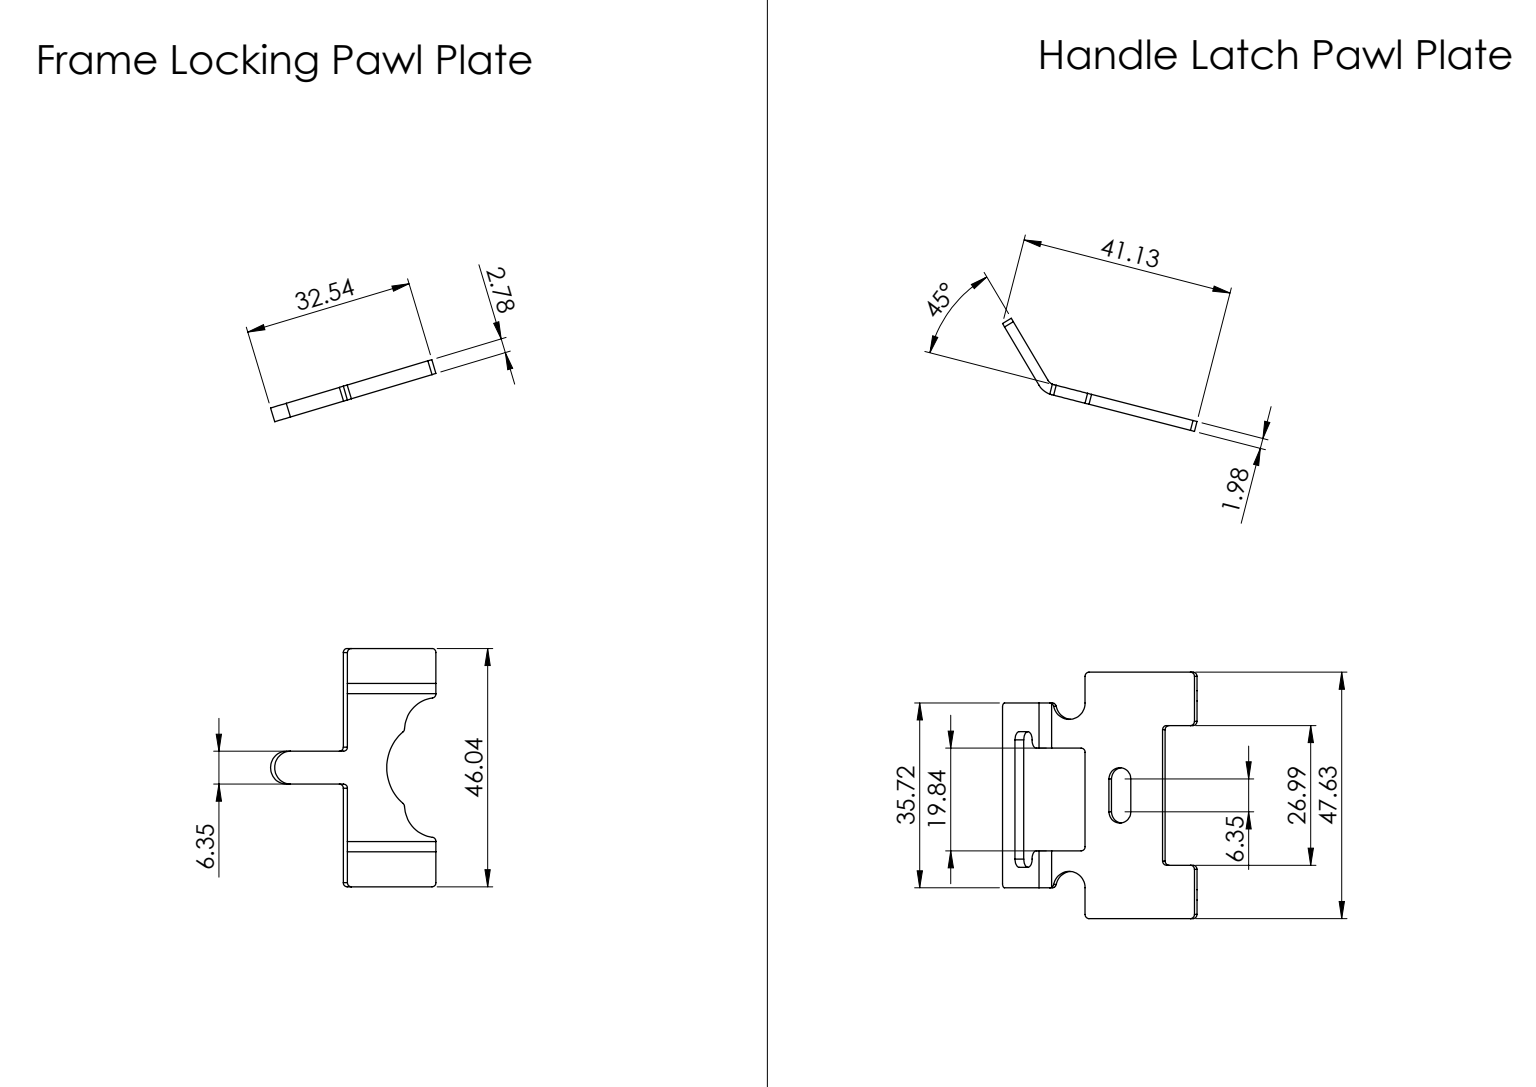
ISO-10303-21;
HEADER;
FILE_DESCRIPTION (('STEP AP214'),
    '1' );
FILE_NAME ('Handle Latch Pawl Plate.step',
    '2026-10-09T14:10:49',
    ( '' ),
    ( '' ),
    'SwSTEP 2.0',
    'SolidWorks 2026',
    '' );
FILE_SCHEMA (( 'AUTOMOTIVE_DESIGN' ));
ENDSEC;

DATA;
#10=CARTESIAN_POINT ( 'NONE',  ( 24.26606285357373594, 2.770822500000000854, -16.92219937337620195 ) ) ;
#13=VECTOR ( 'NONE', #12201, 1000.000000000000000 ) ;
#33=SHAPE_REPRESENTATION_RELATIONSHIP ( 'NONE' , 'NONE' ,  #560, #17207 ) ;
#39=CARTESIAN_POINT ( 'NONE',  ( -0.5435003404963313356, 2.373947500000000765, -25.80650133522849998 ) ) ;
#48=DIRECTION ( 'NONE',  ( 0.000000000000000000, -1.000000000000000000, 0.000000000000000000 ) ) ;
#49=ORIENTED_EDGE ( 'NONE', *, *, #10493, .T. ) ;
#66=ORIENTED_EDGE ( 'NONE', *, *, #20020, .T. ) ;
#83=EDGE_CURVE ( 'NONE', #6123, #21755, #12204, .T. ) ;
#96=DIRECTION ( 'NONE',  ( 0.000000000000000000, 1.000000000000000000, 0.000000000000000000 ) ) ;
#99=VECTOR ( 'NONE', #5317, 1000.000000000000114 ) ;
#111=DIRECTION ( 'NONE',  ( 0.2490110332224850509, 0.000000000000000000, -0.9685006480810792739 ) ) ;
#157=EDGE_CURVE ( 'NONE', #13662, #8452, #17280, .T. ) ;
#167=ADVANCED_FACE ( 'NONE', ( #2245 ), #15977, .T. ) ;
#183=AXIS2_PLACEMENT_3D ( 'NONE', #21265, #19500, #6119 ) ;
#192=CARTESIAN_POINT ( 'NONE',  ( 1.416441012474747074, 34.09397655050049991, -20.74814719358345627 ) ) ;
#195=DIRECTION ( 'NONE',  ( 0.000000000000000000, 1.000000000000000000, 0.000000000000000000 ) ) ;
#203=EDGE_CURVE ( 'NONE', #6199, #19184, #15619, .T. ) ;
#215=CARTESIAN_POINT ( 'NONE',  ( 4.520836821130160388, 5.548947500000001476, -5.476444653012091379 ) ) ;
#222=PLANE ( 'NONE',  #19482 ) ;
#237=EDGE_CURVE ( 'NONE', #10280, #1619, #6209, .T. ) ;
#244=DIRECTION ( 'NONE',  ( 0.8609107660235850723, 0.000000000000000000, -0.5087559856598092844 ) ) ;
#263=ORIENTED_EDGE ( 'NONE', *, *, #13066, .F. ) ;
#272=EDGE_CURVE ( 'NONE', #13945, #11658, #11090, .T. ) ;
#300=DIRECTION ( 'NONE',  ( -0.5087559856598092844, -0.000000000000000000, -0.8609107660235850723 ) ) ;
#308=FACE_OUTER_BOUND ( 'NONE', #12169, .T. ) ;
#318=ORIENTED_EDGE ( 'NONE', *, *, #7660, .F. ) ;
#328=DIRECTION ( 'NONE',  ( -0.2490110332224850509, 0.000000000000000000, 0.9685006480810792739 ) ) ;
#361=CARTESIAN_POINT ( 'NONE',  ( 14.73791976308111451, 13.08957250000000094, -17.32306410839158772 ) ) ;
#372=AXIS2_PLACEMENT_3D ( 'NONE', #2270, #15784, #5467 ) ;
#399=AXIS2_PLACEMENT_3D ( 'NONE', #8708, #17541, #7472 ) ;
#408=CARTESIAN_POINT ( 'NONE',  ( 1.923689137428217455, -0.9589899600121986056, -20.61772871637841220 ) ) ;
#410=VECTOR ( 'NONE', #17472, 1000.000000000000114 ) ;
#415=CARTESIAN_POINT ( 'NONE',  ( -6.268352501591477832, 33.32892749999999893, -35.49402737582407497 ) ) ;
#420=VECTOR ( 'NONE', #6179, 1000.000000000000114 ) ;
#425=EDGE_LOOP ( 'NONE', ( #3626, #10707, #4614, #14152, #12802, #17035 ) ) ;
#431=VECTOR ( 'NONE', #2432, 1000.000000000000114 ) ;
#435=CARTESIAN_POINT ( 'NONE',  ( 28.87608719841374949, 1.975802500000001904, -15.73691681567849976 ) ) ;
#457=ORIENTED_EDGE ( 'NONE', *, *, #18854, .F. ) ;
#462=AXIS2_PLACEMENT_3D ( 'NONE', #21471, #19700, #9852 ) ;
#474=DIRECTION ( 'NONE',  ( 0.2490110332224850231, 0.000000000000000000, -0.9685006480810791629 ) ) ;
#475=CARTESIAN_POINT ( 'NONE',  ( 29.64606458365116737, -7.547927499999999235, -15.53894806404596096 ) ) ;
#478=EDGE_CURVE ( 'NONE', #18112, #12175, #19125, .T. ) ;
#480=ORIENTED_EDGE ( 'NONE', *, *, #17479, .T. ) ;
#490=VERTEX_POINT ( 'NONE', #7825 ) ;
#492=EDGE_CURVE ( 'NONE', #3590, #2498, #6272, .T. ) ;
#508=CARTESIAN_POINT ( 'NONE',  ( 19.07578797920377411, 34.51447250000000366, -18.25667004382573566 ) ) ;
#510=FACE_OUTER_BOUND ( 'NONE', #6893, .T. ) ;
#513=VERTEX_POINT ( 'NONE', #11150 ) ;
#514=DIRECTION ( 'NONE',  ( -0.9685006480810792739, 0.000000000000000000, -0.2490110332224850509 ) ) ;
#517=CARTESIAN_POINT ( 'NONE',  ( 1.670997140563193373, 34.12394749999999988, -22.76294857149378714 ) ) ;
#526=CARTESIAN_POINT ( 'NONE',  ( 1.998220421679061776, 25.39269750000000059, -22.64748046904500356 ) ) ;
#547=DIRECTION ( 'NONE',  ( 0.000000000000000000, 1.000000000000000000, 0.000000000000000000 ) ) ;
#560=SHAPE_REPRESENTATION ( 'Handle Latch Pawl Plate', ( #2234 ), #14439 ) ;
#565=PLANE ( 'NONE',  #6360 ) ;
#578=CARTESIAN_POINT ( 'NONE',  ( -5.536601939709260733, 3.961447500000001565, -30.39452380949970944 ) ) ;
#593=AXIS2_PLACEMENT_3D ( 'NONE', #12095, #15316, #1903 ) ;
#594=CARTESIAN_POINT ( 'NONE',  ( -6.268352501600194415, -1.265494433635971250, -35.49402737582123990 ) ) ;
#631=ORIENTED_EDGE ( 'NONE', *, *, #14864, .T. ) ;
#635=CARTESIAN_POINT ( 'NONE',  ( 7.735533989518945219, 5.548947500000001476, -21.17236077523805449 ) ) ;
#645=VECTOR ( 'NONE', #6896, 1000.000000000000114 ) ;
#647=CARTESIAN_POINT ( 'NONE',  ( 19.07578797920376701, -3.966527499999997097, -18.25667004382573921 ) ) ;
#663=ORIENTED_EDGE ( 'NONE', *, *, #15860, .F. ) ;
#670=CARTESIAN_POINT ( 'NONE',  ( 1.776692311944953584, 34.12394749999999988, -22.71488278333200839 ) ) ;
#720=CIRCLE ( 'NONE', #9536, 0.7950200000000005041 ) ;
#727=ORIENTED_EDGE ( 'NONE', *, *, #2466, .F. ) ;
#732=LINE ( 'NONE', #7593, #11396 ) ;
#750=EDGE_LOOP ( 'NONE', ( #6315, #10700, #9277, #2077, #19066, #6524 ) ) ;
#754=AXIS2_PLACEMENT_3D ( 'NONE', #7235, #13993, #4124 ) ;
#762=ADVANCED_FACE ( 'NONE', ( #16785 ), #13268, .T. ) ;
#788=AXIS2_PLACEMENT_3D ( 'NONE', #5490, #4369, #1956 ) ;
#794=DIRECTION ( 'NONE',  ( -0.000000000000000000, 1.000000000000000000, 0.000000000000000000 ) ) ;
#805=VECTOR ( 'NONE', #14773, 1000.000000000000114 ) ;
#808=EDGE_LOOP ( 'NONE', ( #8099, #12394, #12847, #19398, #3996, #13078 ) ) ;
#839=DIRECTION ( 'NONE',  ( 0.8558687090795832342, 0.000000000000000000, -0.5171931484643309540 ) ) ;
#871=CIRCLE ( 'NONE', #6171, 3.174999999999998490 ) ;
#875=CARTESIAN_POINT ( 'NONE',  ( 2.492193568723835462, -69.63187750000000165, -24.56873394466936134 ) ) ;
#879=CARTESIAN_POINT ( 'NONE',  ( -1.427050033073577806, 5.548947500000001476, -23.44038945102687066 ) ) ;
#884=ORIENTED_EDGE ( 'NONE', *, *, #3946, .T. ) ;
#892=FACE_OUTER_BOUND ( 'NONE', #17084, .T. ) ;
#903=CARTESIAN_POINT ( 'NONE',  ( -23.36909032872569014, 3.961447500000001565, -10.47372115209112842 ) ) ;
#911=EDGE_LOOP ( 'NONE', ( #2038, #5013, #2441, #3955 ) ) ;
#942=DIRECTION ( 'NONE',  ( 0.000000000000000000, -1.000000000000000000, 0.000000000000000000 ) ) ;
#946=PLANE ( 'NONE',  #19198 ) ;
#992=EDGE_CURVE ( 'NONE', #20634, #7630, #3840, .T. ) ;
#999=CARTESIAN_POINT ( 'NONE',  ( 28.38195592936287781, -6.752907499999998286, -13.81504834214261024 ) ) ;
#1000=DIRECTION ( 'NONE',  ( -0.000000000000000000, 1.000000000000000000, 0.000000000000000000 ) ) ;
#1001=DIRECTION ( 'NONE',  ( 0.2490110332224850231, 0.000000000000000000, -0.9685006480810791629 ) ) ;
#1013=VECTOR ( 'NONE', #20361, 1000.000000000000114 ) ;
#1047=ORIENTED_EDGE ( 'NONE', *, *, #11652, .T. ) ;
#1048=LINE ( 'NONE', #21490, #15598 ) ;
#1071=DIRECTION ( 'NONE',  ( 0.9685006480810790519, 0.000000000000000000, 0.2490110332224857170 ) ) ;
#1091=DIRECTION ( 'NONE',  ( 0.000000000000000000, 1.000000000000000000, 0.000000000000000000 ) ) ;
#1093=DIRECTION ( 'NONE',  ( -0.9685006480810791629, 0.000000000000000000, -0.2490110332224850231 ) ) ;
#1096=VERTEX_POINT ( 'NONE', #4892 ) ;
#1134=ORIENTED_EDGE ( 'NONE', *, *, #19533, .F. ) ;
#1150=CARTESIAN_POINT ( 'NONE',  ( 28.38195592936287781, 2.770822500000000854, -13.81504834214261024 ) ) ;
#1154=DIRECTION ( 'NONE',  ( -0.8558687090795832342, 0.000000000000000000, 0.5171931484643309540 ) ) ;
#1180=CARTESIAN_POINT ( 'NONE',  ( 15.23205103213198441, 13.08957250000000094, -19.24493258192747902 ) ) ;
#1194=EDGE_LOOP ( 'NONE', ( #3150, #13135, #19731, #16444 ) ) ;
#1196=DIRECTION ( 'NONE',  ( -0.8609107660235849613, 0.000000000000000000, 0.5087559856598092844 ) ) ;
#1200=DIRECTION ( 'NONE',  ( -0.2490110332224850509, 0.000000000000000000, 0.9685006480810792739 ) ) ;
#1216=VERTEX_POINT ( 'NONE', #20126 ) ;
#1220=EDGE_CURVE ( 'NONE', #9160, #4533, #11757, .T. ) ;
#1267=( NAMED_UNIT ( * ) PLANE_ANGLE_UNIT ( ) SI_UNIT ( $, .RADIAN. ) );
#1281=CARTESIAN_POINT ( 'NONE',  ( -6.268352501604232963, 33.79463943363963807, -35.49402737582801848 ) ) ;
#1282=DIRECTION ( 'NONE',  ( -0.5087559856598092844, 0.000000000000000000, -0.8609107660235849613 ) ) ;
#1290=ADVANCED_FACE ( 'NONE', ( #17049 ), #1896, .T. ) ;
#1295=VERTEX_POINT ( 'NONE', #13752 ) ;
#1336=ADVANCED_FACE ( 'NONE', ( #17716 ), #15964, .T. ) ;
#1355=EDGE_CURVE ( 'NONE', #13546, #14729, #6108, .T. ) ;
#1371=AXIS2_PLACEMENT_3D ( 'NONE', #14359, #9464, #21074 ) ;
#1372=ORIENTED_EDGE ( 'NONE', *, *, #1935, .T. ) ;
#1407=VECTOR ( 'NONE', #1001, 1000.000000000000114 ) ;
#1436=CARTESIAN_POINT ( 'NONE',  ( 9.275488759993784527, 39.28205249999999893, -20.77642327197297689 ) ) ;
#1438=DIRECTION ( 'NONE',  ( -0.3393000355767771259, 0.000000000000000000, 0.9406782052634140578 ) ) ;
#1472=ORIENTED_EDGE ( 'NONE', *, *, #18070, .T. ) ;
#1473=DIRECTION ( 'NONE',  ( 0.000000000000000000, -1.000000000000000000, 0.000000000000000000 ) ) ;
#1480=VERTEX_POINT ( 'NONE', #4310 ) ;
#1484=CIRCLE ( 'NONE', #3603, 1.983740000000000503 ) ;
#1494=CARTESIAN_POINT ( 'NONE',  ( 28.87608719841374949, 29.75832250000000201, -15.73691681567849976 ) ) ;
#1496=VECTOR ( 'NONE', #10087, 1000.000000000000114 ) ;
#1506=DIRECTION ( 'NONE',  ( 0.2490110332224850509, 0.000000000000000000, -0.9685006480810792739 ) ) ;
#1537=ADVANCED_FACE ( 'NONE', ( #4632 ), #2983, .T. ) ;
#1541=ORIENTED_EDGE ( 'NONE', *, *, #4537, .F. ) ;
#1560=EDGE_LOOP ( 'NONE', ( #19520, #15225, #14345, #9159, #6722, #1134 ) ) ;
#1579=LINE ( 'NONE', #11435, #21377 ) ;
#1585=PLANE ( 'NONE',  #593 ) ;
#1601=DIRECTION ( 'NONE',  ( -0.9685006480810791629, 0.000000000000000000, -0.2490110332224850231 ) ) ;
#1612=ORIENTED_EDGE ( 'NONE', *, *, #3894, .T. ) ;
#1619=VERTEX_POINT ( 'NONE', #14609 ) ;
#1632=VERTEX_POINT ( 'NONE', #6178 ) ;
#1645=CARTESIAN_POINT ( 'NONE',  ( -7.949728765564807453, 33.79463943364264367, -34.47798802950575237 ) ) ;
#1646=DIRECTION ( 'NONE',  ( 0.000000000000000000, -1.000000000000000000, 0.000000000000000000 ) ) ;
#1649=CIRCLE ( 'NONE', #18962, 3.970020000000001215 ) ;
#1665=DIRECTION ( 'NONE',  ( -0.5087559856598092844, 0.000000000000000000, -0.8609107660235849613 ) ) ;
#1717=CARTESIAN_POINT ( 'NONE',  ( 11.24737647850577993, 19.43957250000000059, -3.746985211334052046 ) ) ;
#1721=VERTEX_POINT ( 'NONE', #6934 ) ;
#1723=DIRECTION ( 'NONE',  ( 0.000000000000000000, 1.000000000000000000, 0.000000000000000000 ) ) ;
#1740=CARTESIAN_POINT ( 'NONE',  ( 24.26606285357373594, 29.75832250000000201, -16.92219937337620195 ) ) ;
#1757=ORIENTED_EDGE ( 'NONE', *, *, #17479, .F. ) ;
#1762=VERTEX_POINT ( 'NONE', #20081 ) ;
#1766=ORIENTED_EDGE ( 'NONE', *, *, #20682, .F. ) ;
#1782=CARTESIAN_POINT ( 'NONE',  ( 0.2641497867371597752, 26.98019749999999917, -24.43980549416641068 ) ) ;
#1785=B_SPLINE_CURVE_WITH_KNOTS ( 'NONE', 3,
 ( #10743, #10628, #670, #19132 ),
 .UNSPECIFIED., .F., .F.,
 ( 4, 4 ),
 ( 0.000000000000000000, 1.000000000000000000 ),
 .UNSPECIFIED. ) ;
#1804=LINE ( 'NONE', #18606, #19796 ) ;
#1809=ORIENTED_EDGE ( 'NONE', *, *, #492, .F. ) ;
#1840=ORIENTED_EDGE ( 'NONE', *, *, #2050, .F. ) ;
#1864=DIRECTION ( 'NONE',  ( -0.8609107660235848503, 0.000000000000000000, 0.5087559856598096175 ) ) ;
#1865=EDGE_LOOP ( 'NONE', ( #727, #19010, #8001, #1904 ) ) ;
#1869=CARTESIAN_POINT ( 'NONE',  ( 2.520748753591570690, 102.1610225000000014, -24.56335908395234924 ) ) ;
#1874=CARTESIAN_POINT ( 'NONE',  ( -3.042350287543033716, 3.961447500000001565, -26.17378113315171007 ) ) ;
#1875=DIRECTION ( 'NONE',  ( 0.000000000000000000, 1.000000000000000000, 0.000000000000000000 ) ) ;
#1884=CARTESIAN_POINT ( 'NONE',  ( -6.268352501591477832, -7.547927499999999235, -35.49402737582407497 ) ) ;
#1896=PLANE ( 'NONE',  #9972 ) ;
#1903=DIRECTION ( 'NONE',  ( 0.000000000000000000, 1.000000000000000000, 0.000000000000000000 ) ) ;
#1904=ORIENTED_EDGE ( 'NONE', *, *, #10523, .T. ) ;
#1935=EDGE_CURVE ( 'NONE', #19764, #15380, #18870, .T. ) ;
#1938=ORIENTED_EDGE ( 'NONE', *, *, #10853, .F. ) ;
#1952=CARTESIAN_POINT ( 'NONE',  ( 23.77193158452286781, 28.96330250000000461, -15.00033089984030887 ) ) ;
#1956=DIRECTION ( 'NONE',  ( 0.000000000000000000, 1.000000000000000000, 0.000000000000000000 ) ) ;
#1957=DIRECTION ( 'NONE',  ( 0.2490110332224850509, 0.000000000000000000, -0.9685006480810792739 ) ) ;
#1962=ORIENTED_EDGE ( 'NONE', *, *, #7537, .T. ) ;
#1981=VERTEX_POINT ( 'NONE', #15914 ) ;
#2019=DIRECTION ( 'NONE',  ( 0.2490110332224850509, 0.000000000000000000, -0.9685006480810792739 ) ) ;
#2038=ORIENTED_EDGE ( 'NONE', *, *, #2764, .T. ) ;
#2050=EDGE_CURVE ( 'NONE', #21656, #4533, #12134, .T. ) ;
#2061=DIRECTION ( 'NONE',  ( 0.5087559856598092844, 0.000000000000000000, 0.8609107660235849613 ) ) ;
#2077=ORIENTED_EDGE ( 'NONE', *, *, #5527, .F. ) ;
#2078=EDGE_CURVE ( 'NONE', #21155, #5628, #13555, .T. ) ;
#2097=ORIENTED_EDGE ( 'NONE', *, *, #203, .F. ) ;
#2119=CARTESIAN_POINT ( 'NONE',  ( 29.64606458365116737, 34.51447250000000366, -15.53894806404596096 ) ) ;
#2125=CARTESIAN_POINT ( 'NONE',  ( 29.64606458365116737, -6.752907499999998286, -15.53894806404596096 ) ) ;
#2157=ORIENTED_EDGE ( 'NONE', *, *, #21610, .F. ) ;
#2175=CIRCLE ( 'NONE', #10306, 1.983739999999997616 ) ;
#2180=CARTESIAN_POINT ( 'NONE',  ( 29.15193331460030279, 30.55334249999999940, -13.61707959051006966 ) ) ;
#2186=AXIS2_PLACEMENT_3D ( 'NONE', #17579, #18897, #17365 ) ;
#2192=ORIENTED_EDGE ( 'NONE', *, *, #7383, .T. ) ;
#2223=FACE_OUTER_BOUND ( 'NONE', #2461, .T. ) ;
#2234=AXIS2_PLACEMENT_3D ( 'NONE', #14022, #2275, #17644 ) ;
#2239=EDGE_CURVE ( 'NONE', #20753, #11503, #4571, .T. ) ;
#2245=FACE_OUTER_BOUND ( 'NONE', #13627, .T. ) ;
#2250=CARTESIAN_POINT ( 'NONE',  ( 1.291462649553455133, -1.594802499999998124, -20.78637864442906746 ) ) ;
#2263=CARTESIAN_POINT ( 'NONE',  ( 0.7843704457339527591, 25.39269750000000059, -23.55949434567611078 ) ) ;
#2266=AXIS2_PLACEMENT_3D ( 'NONE', #19432, #11373, #9591 ) ;
#2270=CARTESIAN_POINT ( 'NONE',  ( -14.17069798364451927, -1.594802499999999013, -10.28222191653059170 ) ) ;
#2275=DIRECTION ( 'NONE',  ( 0.000000000000000000, 0.000000000000000000, 1.000000000000000000 ) ) ;
#2289=CARTESIAN_POINT ( 'NONE',  ( 2.492193568723835462, -69.63187750000000165, -24.56873394466936134 ) ) ;
#2291=CARTESIAN_POINT ( 'NONE',  ( 1.532169971477637782, 34.03012968715594866, -20.71839214105750315 ) ) ;
#2296=ORIENTED_EDGE ( 'NONE', *, *, #6544, .F. ) ;
#2298=VERTEX_POINT ( 'NONE', #14868 ) ;
#2308=DIRECTION ( 'NONE',  ( -0.9685006480810790519, 0.000000000000000000, -0.2490110332224857170 ) ) ;
#2310=FACE_OUTER_BOUND ( 'NONE', #21323, .T. ) ;
#2318=PLANE ( 'NONE',  #21251 ) ;
#2376=VECTOR ( 'NONE', #10947, 1000.000000000000000 ) ;
#2432=DIRECTION ( 'NONE',  ( -0.5087559856598092844, 0.000000000000000000, -0.8609107660235849613 ) ) ;
#2435=ORIENTED_EDGE ( 'NONE', *, *, #21472, .F. ) ;
#2438=DIRECTION ( 'NONE',  ( 0.5087559856598092844, 0.000000000000000000, 0.8609107660235849613 ) ) ;
#2441=ORIENTED_EDGE ( 'NONE', *, *, #5568, .T. ) ;
#2443=AXIS2_PLACEMENT_3D ( 'NONE', #4092, #7521, #10832 ) ;
#2461=EDGE_LOOP ( 'NONE', ( #884, #4206, #14313, #10118, #4181, #10108, #18999, #16892, #15929, #1766, #8567, #19717, #16820, #19420, #14827, #10153, #7652, #7601, #20757, #17660, #1472, #1047, #8293, #7481, #4823, #18978, #17213, #16162 ) ) ;
#2466=EDGE_CURVE ( 'NONE', #21748, #1981, #7554, .T. ) ;
#2495=VERTEX_POINT ( 'NONE', #9826 ) ;
#2498=VERTEX_POINT ( 'NONE', #19892 ) ;
#2510=DIRECTION ( 'NONE',  ( 0.9685006480810790519, 0.000000000000000000, 0.2490110332224857170 ) ) ;
#2523=AXIS2_PLACEMENT_3D ( 'NONE', #16109, #9012, #7687 ) ;
#2526=ORIENTED_EDGE ( 'NONE', *, *, #18854, .T. ) ;
#2541=CARTESIAN_POINT ( 'NONE',  ( -1.629142294184690698, 34.12394749999999988, -7.057664713974870274 ) ) ;
#2552=DIRECTION ( 'NONE',  ( 0.9685006480810793850, 0.000000000000000000, 0.2490110332224848011 ) ) ;
#2558=VECTOR ( 'NONE', #21534, 1000.000000000000000 ) ;
#2569=DIRECTION ( 'NONE',  ( 0.000000000000000000, 1.000000000000000000, 0.000000000000000000 ) ) ;
#2577=VERTEX_POINT ( 'NONE', #8385 ) ;
#2598=EDGE_CURVE ( 'NONE', #17189, #7442, #7339, .T. ) ;
#2605=VECTOR ( 'NONE', #10573, 1000.000000000000000 ) ;
#2627=DIRECTION ( 'NONE',  ( 0.2490110332224850509, 0.000000000000000000, -0.9685006480810792739 ) ) ;
#2639=EDGE_LOOP ( 'NONE', ( #4484, #9676, #15711, #14242 ) ) ;
#2653=LINE ( 'NONE', #16150, #6790 ) ;
#2663=VECTOR ( 'NONE', #20289, 1000.000000000000000 ) ;
#2685=ORIENTED_EDGE ( 'NONE', *, *, #18562, .F. ) ;
#2718=ORIENTED_EDGE ( 'NONE', *, *, #237, .F. ) ;
#2756=PRESENTATION_STYLE_ASSIGNMENT (( #12949 ) ) ;
#2757=ORIENTED_EDGE ( 'NONE', *, *, #13924, .F. ) ;
#2764=EDGE_CURVE ( 'NONE', #8452, #12517, #10390, .T. ) ;
#2765=ORIENTED_EDGE ( 'NONE', *, *, #19882, .T. ) ;
#2769=AXIS2_PLACEMENT_3D ( 'NONE', #10291, #10413, #18685 ) ;
#2772=DIRECTION ( 'NONE',  ( 0.2490110332224850231, 0.000000000000000000, -0.9685006480810791629 ) ) ;
#2788=EDGE_CURVE ( 'NONE', #1096, #20725, #5083, .T. ) ;
#2791=EDGE_CURVE ( 'NONE', #8452, #7807, #20762, .T. ) ;
#2796=VECTOR ( 'NONE', #4237, 1000.000000000000114 ) ;
#2799=CARTESIAN_POINT ( 'NONE',  ( 24.26606285357373594, 2.770822500000000854, -16.92219937337620195 ) ) ;
#2815=ORIENTED_EDGE ( 'NONE', *, *, #14864, .F. ) ;
#2837=VECTOR ( 'NONE', #474, 1000.000000000000114 ) ;
#2842=ADVANCED_FACE ( 'NONE', ( #12165 ), #5623, .F. ) ;
#2864=AXIS2_PLACEMENT_3D ( 'NONE', #5931, #9034, #1071 ) ;
#2871=ORIENTED_EDGE ( 'NONE', *, *, #992, .F. ) ;
#2883=AXIS2_PLACEMENT_3D ( 'NONE', #361, #12308, #10651 ) ;
#2898=DIRECTION ( 'NONE',  ( 0.000000000000000000, 1.000000000000000000, 0.000000000000000000 ) ) ;
#2903=ORIENTED_EDGE ( 'NONE', *, *, #20412, .T. ) ;
#2933=LINE ( 'NONE', #9660, #12813 ) ;
#2943=VERTEX_POINT ( 'NONE', #13832 ) ;
#2944=AXIS2_PLACEMENT_3D ( 'NONE', #1782, #12081, #20447 ) ;
#2951=AXIS2_PLACEMENT_3D ( 'NONE', #11235, #14800, #2510 ) ;
#2962=ORIENTED_EDGE ( 'NONE', *, *, #11927, .F. ) ;
#2968=AXIS2_PLACEMENT_3D ( 'NONE', #8717, #12385, #2308 ) ;
#2973=AXIS2_PLACEMENT_3D ( 'NONE', #19298, #7264, #12679 ) ;
#2979=DIRECTION ( 'NONE',  ( 0.2490110332224850231, 0.000000000000000000, -0.9685006480810791629 ) ) ;
#2982=ORIENTED_EDGE ( 'NONE', *, *, #5220, .F. ) ;
#2983=CYLINDRICAL_SURFACE ( 'NONE', #7522, 0.7950200000000001710 ) ;
#2994=VERTEX_POINT ( 'NONE', #6273 ) ;
#3000=DIRECTION ( 'NONE',  ( 0.000000000000000000, -1.000000000000000000, 0.000000000000000000 ) ) ;
#3012=ORIENTED_EDGE ( 'NONE', *, *, #478, .T. ) ;
#3039=ORIENTED_EDGE ( 'NONE', *, *, #13022, .F. ) ;
#3058=CARTESIAN_POINT ( 'NONE',  ( -6.268352501591477832, 33.32892749999999893, -35.49402737582407497 ) ) ;
#3075=ORIENTED_EDGE ( 'NONE', *, *, #7315, .F. ) ;
#3088=CARTESIAN_POINT ( 'NONE',  ( 1.998220421679061776, -1.515722362770699494, -22.64748046904500356 ) ) ;
#3111=VERTEX_POINT ( 'NONE', #7826 ) ;
#3119=CARTESIAN_POINT ( 'NONE',  ( 7.735533989518945219, 5.548947500000001476, -21.17236077523805449 ) ) ;
#3122=DIRECTION ( 'NONE',  ( 0.000000000000000000, -1.000000000000000000, 0.000000000000000000 ) ) ;
#3150=ORIENTED_EDGE ( 'NONE', *, *, #11028, .T. ) ;
#3152=ORIENTED_EDGE ( 'NONE', *, *, #21472, .T. ) ;
#3158=LINE ( 'NONE', #15016, #5901 ) ;
#3181=CARTESIAN_POINT ( 'NONE',  ( 24.36723594150488026, 30.55334249999999940, 1.799757394719970982 ) ) ;
#3183=VECTOR ( 'NONE', #48, 1000.000000000000000 ) ;
#3198=DIRECTION ( 'NONE',  ( -0.2490110332224849676, 0.000000000000000000, 0.9685006480810792739 ) ) ;
#3206=DIRECTION ( 'NONE',  ( -0.2490110332224850509, 0.000000000000000000, 0.9685006480810792739 ) ) ;
#3207=AXIS2_PLACEMENT_3D ( 'NONE', #5858, #16163, #5960 ) ;
#3228=CIRCLE ( 'NONE', #20150, 1.983740000000001391 ) ;
#3230=LINE ( 'NONE', #3119, #15881 ) ;
#3231=CARTESIAN_POINT ( 'NONE',  ( 1.169308704210513694, 33.32892749999999893, -20.81168733838920915 ) ) ;
#3245=DIRECTION ( 'NONE',  ( -0.8609107660235849613, 0.000000000000000000, 0.5087559856598092844 ) ) ;
#3248=DIRECTION ( 'NONE',  ( 0.000000000000000000, 1.000000000000000000, 0.000000000000000000 ) ) ;
#3267=AXIS2_PLACEMENT_3D ( 'NONE', #16888, #1957, #11705 ) ;
#3269=DIRECTION ( 'NONE',  ( 0.2490110332224850231, 0.000000000000000000, -0.9685006480810791629 ) ) ;
#3273=MECHANICAL_DESIGN_GEOMETRIC_PRESENTATION_REPRESENTATION('',(#11042),#7510);
#3275=CARTESIAN_POINT ( 'NONE',  ( 1.998220421679061776, 5.548947500000001476, -22.64748046904500356 ) ) ;
#3288=DIRECTION ( 'NONE',  ( -0.9685006480810791629, 0.000000000000000000, -0.2490110332224850509 ) ) ;
#3295=EDGE_LOOP ( 'NONE', ( #17508, #19503, #2757, #7196 ) ) ;
#3306=CARTESIAN_POINT ( 'NONE',  ( 17.34610635302146164, 19.43957250000000059, -18.70138818597152053 ) ) ;
#3328=FACE_OUTER_BOUND ( 'NONE', #7245, .T. ) ;
#3340=CARTESIAN_POINT ( 'NONE',  ( -7.949728765565600597, -0.7997824999999986195, -34.47798802950714503 ) ) ;
#3342=ORIENTED_EDGE ( 'NONE', *, *, #18833, .F. ) ;
#3360=CARTESIAN_POINT ( 'NONE',  ( -1.351150467732365579, 28.56769750000000130, -27.17319717629097653 ) ) ;
#3375=LINE ( 'NONE', #17178, #645 ) ;
#3390=ORIENTED_EDGE ( 'NONE', *, *, #5399, .F. ) ;
#3399=CARTESIAN_POINT ( 'NONE',  ( 24.26606285357373594, 29.75832250000000201, -16.92219937337620195 ) ) ;
#3406=VERTEX_POINT ( 'NONE', #14433 ) ;
#3409=DIRECTION ( 'NONE',  ( -0.2490110332224848289, 0.000000000000000000, 0.9685006480810792739 ) ) ;
#3426=PLANE ( 'NONE',  #15712 ) ;
#3427=DIRECTION ( 'NONE',  ( 0.8609107660235850723, 0.000000000000000000, -0.5087559856598092844 ) ) ;
#3438=ORIENTED_EDGE ( 'NONE', *, *, #18458, .F. ) ;
#3445=CYLINDRICAL_SURFACE ( 'NONE', #2769, 3.970020000000001215 ) ;
#3484=EDGE_CURVE ( 'NONE', #1216, #16869, #14872, .T. ) ;
#3486=EDGE_LOOP ( 'NONE', ( #10195, #2685, #263, #12752 ) ) ;
#3501=DIRECTION ( 'NONE',  ( -0.2490110332224850231, 0.000000000000000000, 0.9685006480810791629 ) ) ;
#3514=DIRECTION ( 'NONE',  ( 0.000000000000000000, -1.000000000000000000, 0.000000000000000000 ) ) ;
#3544=VECTOR ( 'NONE', #17324, 1000.000000000000114 ) ;
#3550=DIRECTION ( 'NONE',  ( 0.000000000000000000, 1.000000000000000000, 0.000000000000000000 ) ) ;
#3567=DIRECTION ( 'NONE',  ( 0.8609107660235849613, 0.000000000000000000, -0.5087559856598092844 ) ) ;
#3581=CARTESIAN_POINT ( 'NONE',  ( -7.949728765565600597, -0.7997824999999986195, -34.47798802950714503 ) ) ;
#3590=VERTEX_POINT ( 'NONE', #3360 ) ;
#3603=AXIS2_PLACEMENT_3D ( 'NONE', #6066, #3514, #3409 ) ;
#3621=CARTESIAN_POINT ( 'NONE',  ( 1.998220421679061776, 34.04486736277070236, -22.64748046904500356 ) ) ;
#3626=ORIENTED_EDGE ( 'NONE', *, *, #7995, .T. ) ;
#3642=EDGE_CURVE ( 'NONE', #20985, #1632, #11500, .T. ) ;
#3649=CYLINDRICAL_SURFACE ( 'NONE', #4762, 3.970020000000001215 ) ;
#3659=DIRECTION ( 'NONE',  ( 0.000000000000000000, -1.000000000000000000, 0.000000000000000000 ) ) ;
#3670=EDGE_CURVE ( 'NONE', #20634, #14970, #10774, .T. ) ;
#3697=EDGE_CURVE ( 'NONE', #6074, #18112, #14957, .T. ) ;
#3716=DIRECTION ( 'NONE',  ( -0.2490110332224850231, 0.000000000000000000, 0.9685006480810791629 ) ) ;
#3726=EDGE_CURVE ( 'NONE', #21188, #16869, #19921, .T. ) ;
#3747=ADVANCED_FACE ( 'NONE', ( #12166 ), #3649, .T. ) ;
#3773=DIRECTION ( 'NONE',  ( -0.8609107660235850723, 0.000000000000000000, 0.5087559856598092844 ) ) ;
#3780=CARTESIAN_POINT ( 'NONE',  ( 29.64606458365116737, -6.752907499999998286, -15.53894806404596096 ) ) ;
#3799=VECTOR ( 'NONE', #11020, 1000.000000000000000 ) ;
#3802=ORIENTED_EDGE ( 'NONE', *, *, #4272, .T. ) ;
#3804=CARTESIAN_POINT ( 'NONE',  ( 1.173720826352361080, -1.594802499999999013, -20.82884779549221577 ) ) ;
#3831=DIRECTION ( 'NONE',  ( 0.2490110332224850231, 0.000000000000000000, -0.9685006480810791629 ) ) ;
#3836=ORIENTED_EDGE ( 'NONE', *, *, #3946, .F. ) ;
#3840=LINE ( 'NONE', #20504, #12824 ) ;
#3849=CARTESIAN_POINT ( 'NONE',  ( -1.351150467732365579, 2.373947500000000765, -27.17319717629097653 ) ) ;
#3860=ADVANCED_FACE ( 'NONE', ( #2310 ), #9266, .F. ) ;
#3866=ADVANCED_FACE ( 'NONE', ( #14377 ), #20996, .T. ) ;
#3868=VECTOR ( 'NONE', #3716, 1000.000000000000114 ) ;
#3877=FACE_OUTER_BOUND ( 'NONE', #7700, .T. ) ;
#3878=LINE ( 'NONE', #15727, #410 ) ;
#3879=DIRECTION ( 'NONE',  ( 0.2490110332224850509, 0.000000000000000000, -0.9685006480810792739 ) ) ;
#3887=FACE_OUTER_BOUND ( 'NONE', #18893, .T. ) ;
#3894=EDGE_CURVE ( 'NONE', #17254, #18451, #871, .T. ) ;
#3923=CIRCLE ( 'NONE', #7106, 0.7950200000000005041 ) ;
#3936=CARTESIAN_POINT ( 'NONE',  ( 13.36143179939526071, 19.43957250000000059, -3.203440815378094886 ) ) ;
#3941=VECTOR ( 'NONE', #20801, 1000.000000000000227 ) ;
#3946=EDGE_CURVE ( 'NONE', #18904, #18859, #10609, .T. ) ;
#3955=ORIENTED_EDGE ( 'NONE', *, *, #2791, .F. ) ;
#3996=ORIENTED_EDGE ( 'NONE', *, *, #19377, .F. ) ;
#3999=AXIS2_PLACEMENT_3D ( 'NONE', #9753, #16516, #17162 ) ;
#4001=DIRECTION ( 'NONE',  ( -0.2490110332224850231, 0.000000000000000000, 0.9685006480810791629 ) ) ;
#4006=CYLINDRICAL_SURFACE ( 'NONE', #16938, 1.587499999999998579 ) ;
#4021=DIRECTION ( 'NONE',  ( 0.000000000000000000, 1.000000000000000000, 0.000000000000000000 ) ) ;
#4029=LINE ( 'NONE', #19376, #8618 ) ;
#4053=CARTESIAN_POINT ( 'NONE',  ( 2.520748753591570690, 5.548947500000001476, -24.56335908395234924 ) ) ;
#4084=DIRECTION ( 'NONE',  ( 0.000000000000000000, 1.000000000000000000, 0.000000000000000000 ) ) ;
#4090=CARTESIAN_POINT ( 'NONE',  ( 28.38195592936287781, 40.07707250000000698, -13.81504834214261024 ) ) ;
#4092=CARTESIAN_POINT ( 'NONE',  ( -2.845411283647486300, 33.32892749999999893, -5.196881601526627925 ) ) ;
#4093=ORIENTED_EDGE ( 'NONE', *, *, #17551, .T. ) ;
#4106=PLANE ( 'NONE',  #6987 ) ;
#4113=CARTESIAN_POINT ( 'NONE',  ( 8.011380105705496746, 6.343967500000000648, -19.05252355006962617 ) ) ;
#4116=CARTESIAN_POINT ( 'NONE',  ( 12.62386444219163373, 13.08957250000000094, -17.86660850434754266 ) ) ;
#4123=ORIENTED_EDGE ( 'NONE', *, *, #10853, .T. ) ;
#4124=DIRECTION ( 'NONE',  ( 0.9488823340533351081, -0.2002559181062070481, 0.2439669719140998283 ) ) ;
#4126=LINE ( 'NONE', #12647, #14824 ) ;
#4150=ORIENTED_EDGE ( 'NONE', *, *, #21680, .F. ) ;
#4181=ORIENTED_EDGE ( 'NONE', *, *, #12897, .T. ) ;
#4185=EDGE_CURVE ( 'NONE', #20863, #16425, #19251, .T. ) ;
#4188=CARTESIAN_POINT ( 'NONE',  ( -4.728951812473551897, 26.98019749999999917, -29.02782796843600011 ) ) ;
#4206=ORIENTED_EDGE ( 'NONE', *, *, #8093, .F. ) ;
#4211=CARTESIAN_POINT ( 'NONE',  ( 17.34610635302146164, 19.43957250000000059, -18.70138818597152053 ) ) ;
#4212=CARTESIAN_POINT ( 'NONE',  ( -0.06046748314524758028, -7.547927499999999235, -21.12787488008327585 ) ) ;
#4229=EDGE_LOOP ( 'NONE', ( #17611, #14707, #2097, #5148 ) ) ;
#4237=DIRECTION ( 'NONE',  ( 0.2490110332224850231, 0.000000000000000000, -0.9685006480810791629 ) ) ;
#4242=( BOUNDED_CURVE ( )  B_SPLINE_CURVE ( 3, ( #3581, #17067, #6674, #20146 ),
 .UNSPECIFIED., .F., .F. ) 
 B_SPLINE_CURVE_WITH_KNOTS ( ( 4, 4 ),
 ( 0.000000000000000000, 1.570796326786294994 ),
 .UNSPECIFIED. ) 
 CURVE ( )  GEOMETRIC_REPRESENTATION_ITEM ( )  RATIONAL_B_SPLINE_CURVE ( ( 1.000000000000000000, 0.8047378541263923157, 0.8047378541263923157, 1.000000000000000000 ) ) 
 REPRESENTATION_ITEM ( '' )  );
#4244=ADVANCED_FACE ( 'NONE', ( #18226 ), #21201, .T. ) ;
#4269=AXIS2_PLACEMENT_3D ( 'NONE', #18071, #11210, #3248 ) ;
#4272=EDGE_CURVE ( 'NONE', #19184, #18464, #10245, .T. ) ;
#4281=CARTESIAN_POINT ( 'NONE',  ( 8.505511374756364873, -6.752907499999998286, -20.97439202360551747 ) ) ;
#4289=VERTEX_POINT ( 'NONE', #17109 ) ;
#4310=CARTESIAN_POINT ( 'NONE',  ( 28.38195592936287781, 29.75832250000000201, -13.81504834214261024 ) ) ;
#4313=SURFACE_SIDE_STYLE ('',( #9710 ) ) ;
#4348=ORIENTED_EDGE ( 'NONE', *, *, #20281, .T. ) ;
#4369=DIRECTION ( 'NONE',  ( 0.2490110332224850509, 0.000000000000000000, -0.9685006480810792739 ) ) ;
#4383=EDGE_LOOP ( 'NONE', ( #2871, #4348, #4906, #480, #6951, #21192 ) ) ;
#4408=VERTEX_POINT ( 'NONE', #3306 ) ;
#4416=CARTESIAN_POINT ( 'NONE',  ( -1.351150467732365579, 28.56769750000000130, -27.17319717629097653 ) ) ;
#4433=DIRECTION ( 'NONE',  ( 0.000000000000000000, -1.000000000000000000, 0.000000000000000000 ) ) ;
#4455=ORIENTED_EDGE ( 'NONE', *, *, #3697, .T. ) ;
#4484=ORIENTED_EDGE ( 'NONE', *, *, #3484, .T. ) ;
#4497=DIRECTION ( 'NONE',  ( -0.8609107660235850723, 0.000000000000000000, 0.5087559856598092844 ) ) ;
#4521=VERTEX_POINT ( 'NONE', #408 ) ;
#4530=DIRECTION ( 'NONE',  ( -0.4139637392816631345, 0.000000000000000000, 0.9102933716994446867 ) ) ;
#4533=VERTEX_POINT ( 'NONE', #1150 ) ;
#4537=EDGE_CURVE ( 'NONE', #20882, #16262, #7780, .T. ) ;
#4538=EDGE_CURVE ( 'NONE', #16037, #2994, #7958, .T. ) ;
#4541=LINE ( 'NONE', #14733, #6353 ) ;
#4549=LINE ( 'NONE', #12865, #9875 ) ;
#4551=CARTESIAN_POINT ( 'NONE',  ( 8.505511374756364873, 39.28205249999999893, -20.97439202360551747 ) ) ;
#4571=LINE ( 'NONE', #7775, #10722 ) ;
#4602=VECTOR ( 'NONE', #3550, 1000.000000000000000 ) ;
#4614=ORIENTED_EDGE ( 'NONE', *, *, #10523, .F. ) ;
#4620=ORIENTED_EDGE ( 'NONE', *, *, #15180, .T. ) ;
#4626=CYLINDRICAL_SURFACE ( 'NONE', #2266, 3.174999999999999378 ) ;
#4632=FACE_OUTER_BOUND ( 'NONE', #8935, .T. ) ;
#4645=CARTESIAN_POINT ( 'NONE',  ( -1.427050033073577806, 25.39269750000000059, -23.44038945102687066 ) ) ;
#4655=CARTESIAN_POINT ( 'NONE',  ( 28.87608719841374949, -7.547927499999999235, -15.73691681567849976 ) ) ;
#4661=CARTESIAN_POINT ( 'NONE',  ( 1.532169971477637782, 25.39269750000000059, -20.71839214105750315 ) ) ;
#4686=DIRECTION ( 'NONE',  ( -0.5087559856598092844, 0.000000000000000000, -0.8609107660235850723 ) ) ;
#4693=EDGE_CURVE ( 'NONE', #8797, #6208, #19818, .T. ) ;
#4719=CARTESIAN_POINT ( 'NONE',  ( -3.845402119898529758, 26.98019749999999917, -31.39393985263922460 ) ) ;
#4744=PRODUCT ( 'Handle Latch Pawl Plate', 'Handle Latch Pawl Plate', '', ( #7336 ) ) ;
#4762=AXIS2_PLACEMENT_3D ( 'NONE', #1869, #6625, #8386 ) ;
#4766=DIRECTION ( 'NONE',  ( 0.9685006480810792739, -0.000000000000000000, 0.2490110332224850509 ) ) ;
#4771=EDGE_CURVE ( 'NONE', #18623, #10280, #1579, .T. ) ;
#4775=DIRECTION ( 'NONE',  ( -0.8609107660235850723, 0.000000000000000000, 0.5087559856598092844 ) ) ;
#4789=ORIENTED_EDGE ( 'NONE', *, *, #18705, .T. ) ;
#4801=DIRECTION ( 'NONE',  ( -0.9685006480810791629, 0.000000000000000000, -0.2490110332224850231 ) ) ;
#4823=ORIENTED_EDGE ( 'NONE', *, *, #19349, .T. ) ;
#4861=VERTEX_POINT ( 'NONE', #5213 ) ;
#4870=EDGE_LOOP ( 'NONE', ( #21436, #318, #12492, #10388 ) ) ;
#4873=DIRECTION ( 'NONE',  ( -0.2490110332224850509, 0.000000000000000000, 0.9685006480810792739 ) ) ;
#4892=CARTESIAN_POINT ( 'NONE',  ( -0.8970842057359728061, 34.12394749999999988, -22.54358764576276286 ) ) ;
#4906=ORIENTED_EDGE ( 'NONE', *, *, #17122, .T. ) ;
#4912=EDGE_CURVE ( 'NONE', #13662, #20882, #6906, .T. ) ;
#4935=ORIENTED_EDGE ( 'NONE', *, *, #6521, .F. ) ;
#4962=VECTOR ( 'NONE', #5043, 1000.000000000000000 ) ;
#4980=ADVANCED_FACE ( 'NONE', ( #15644, #13872 ), #6984, .T. ) ;
#4989=DIRECTION ( 'NONE',  ( 0.9488823340533149020, 0.2002559181063070792, 0.2439669719140961091 ) ) ;
#4999=VECTOR ( 'NONE', #16604, 1000.000000000000114 ) ;
#5000=AXIS2_PLACEMENT_3D ( 'NONE', #13880, #15651, #8352 ) ;
#5010=VECTOR ( 'NONE', #1875, 1000.000000000000000 ) ;
#5013=ORIENTED_EDGE ( 'NONE', *, *, #10687, .T. ) ;
#5015=CARTESIAN_POINT ( 'NONE',  ( 14.73791976308111451, 19.43957250000000059, -17.32306410839158772 ) ) ;
#5041=ORIENTED_EDGE ( 'NONE', *, *, #4693, .F. ) ;
#5043=DIRECTION ( 'NONE',  ( 0.000000000000000000, -1.000000000000000000, 0.000000000000000000 ) ) ;
#5045=CIRCLE ( 'NONE', #3999, 0.7950200000000003930 ) ;
#5076=ORIENTED_EDGE ( 'NONE', *, *, #18241, .T. ) ;
#5083=CIRCLE ( 'NONE', #12872, 3.970020000000002991 ) ;
#5128=DIRECTION ( 'NONE',  ( 0.000000000000000000, -1.000000000000000000, 0.000000000000000000 ) ) ;
#5148=ORIENTED_EDGE ( 'NONE', *, *, #7732, .T. ) ;
#5150=CARTESIAN_POINT ( 'NONE',  ( 28.38195592936287781, 29.75832250000000201, -13.81504834214261024 ) ) ;
#5190=CARTESIAN_POINT ( 'NONE',  ( 8.505511374756364873, -6.752907499999998286, -20.97439202360551747 ) ) ;
#5197=ADVANCED_FACE ( 'NONE', ( #11082 ), #14411, .F. ) ;
#5213=CARTESIAN_POINT ( 'NONE',  ( 7.241402720468077092, 5.548947500000001476, -19.25049230170216319 ) ) ;
#5220=EDGE_CURVE ( 'NONE', #18746, #1762, #15622, .T. ) ;
#5238=ORIENTED_EDGE ( 'NONE', *, *, #14198, .F. ) ;
#5243=VECTOR ( 'NONE', #19413, 1000.000000000000114 ) ;
#5263=CARTESIAN_POINT ( 'NONE',  ( 9.275488759993784527, -6.752907499999998286, -20.77642327197297689 ) ) ;
#5282=EDGE_CURVE ( 'NONE', #4533, #1721, #9734, .T. ) ;
#5288=EDGE_LOOP ( 'NONE', ( #5396, #12812, #11337, #5076 ) ) ;
#5294=EDGE_CURVE ( 'NONE', #12469, #4408, #8878, .T. ) ;
#5317=DIRECTION ( 'NONE',  ( 0.8609107660235849613, 0.000000000000000000, -0.5087559856598092844 ) ) ;
#5325=VECTOR ( 'NONE', #16325, 1000.000000000000114 ) ;
#5362=PLANE ( 'NONE',  #19736 ) ;
#5368=VECTOR ( 'NONE', #7621, 1000.000000000000114 ) ;
#5376=LINE ( 'NONE', #12139, #3544 ) ;
#5396=ORIENTED_EDGE ( 'NONE', *, *, #5294, .T. ) ;
#5399=EDGE_CURVE ( 'NONE', #4289, #10917, #21588, .T. ) ;
#5409=FACE_OUTER_BOUND ( 'NONE', #5851, .T. ) ;
#5433=LINE ( 'NONE', #4116, #2837 ) ;
#5442=CARTESIAN_POINT ( 'NONE',  ( 7.735533989518945219, 25.39269750000000059, -21.17236077523805449 ) ) ;
#5448=CARTESIAN_POINT ( 'NONE',  ( 1.532169971477637782, -1.500984687155947128, -20.71839214105750315 ) ) ;
#5462=ORIENTED_EDGE ( 'NONE', *, *, #11884, .F. ) ;
#5467=DIRECTION ( 'NONE',  ( 0.9685006480810792739, 0.000000000000000000, 0.2490110332224850509 ) ) ;
#5470=DIRECTION ( 'NONE',  ( -0.8609107660235850723, 0.000000000000000000, 0.5087559856598092844 ) ) ;
#5489=DIRECTION ( 'NONE',  ( 0.2490110332224850231, 0.000000000000000000, -0.9685006480810791629 ) ) ;
#5490=CARTESIAN_POINT ( 'NONE',  ( 7.241402720468077092, 24.59767750000000319, -19.25049230170216319 ) ) ;
#5493=EDGE_LOOP ( 'NONE', ( #20747, #8034, #13696, #5588, #16901, #5041, #17997, #21400, #15815, #14066, #20542, #12274, #8699, #1757, #16589, #5238, #18655, #6845, #12571, #11448, #19044, #11895, #12905, #3342 ) ) ;
#5506=ORIENTED_EDGE ( 'NONE', *, *, #12874, .F. ) ;
#5508=DIRECTION ( 'NONE',  ( 0.2490110332224850509, 0.000000000000000000, -0.9685006480810792739 ) ) ;
#5527=EDGE_CURVE ( 'NONE', #11596, #14232, #13960, .T. ) ;
#5534=FACE_OUTER_BOUND ( 'NONE', #13354, .T. ) ;
#5535=VECTOR ( 'NONE', #12022, 1000.000000000000000 ) ;
#5568=EDGE_CURVE ( 'NONE', #11596, #7807, #3878, .T. ) ;
#5584=CIRCLE ( 'NONE', #13372, 0.7950200000000012812 ) ;
#5588=ORIENTED_EDGE ( 'NONE', *, *, #4538, .T. ) ;
#5593=EDGE_CURVE ( 'NONE', #9048, #16262, #2653, .T. ) ;
#5617=VECTOR ( 'NONE', #2061, 1000.000000000000114 ) ;
#5621=EDGE_CURVE ( 'NONE', #1096, #17189, #21001, .T. ) ;
#5623=CYLINDRICAL_SURFACE ( 'NONE', #2968, 0.7950200000000003930 ) ;
#5624=CARTESIAN_POINT ( 'NONE',  ( 5.430521817098937554, 34.12394749999999988, -21.76500205408690647 ) ) ;
#5628=VERTEX_POINT ( 'NONE', #9382 ) ;
#5647=CIRCLE ( 'NONE', #7044, 0.7950200000000000600 ) ;
#5650=LINE ( 'NONE', #10747, #7881 ) ;
#5656=ADVANCED_FACE ( 'NONE', ( #21097 ), #14063, .T. ) ;
#5664=CARTESIAN_POINT ( 'NONE',  ( 0.7843704457339527591, 5.548947500000001476, -23.55949434567611078 ) ) ;
#5667=VERTEX_POINT ( 'NONE', #12605 ) ;
#5688=UNCERTAINTY_MEASURE_WITH_UNIT (LENGTH_MEASURE( 1.000000000000000082E-05 ), #16367, 'distance_accuracy_value', 'NONE');
#5697=PLANE ( 'NONE',  #372 ) ;
#5711=ORIENTED_EDGE ( 'NONE', *, *, #10696, .F. ) ;
#5726=ORIENTED_EDGE ( 'NONE', *, *, #13204, .F. ) ;
#5727=ORIENTED_EDGE ( 'NONE', *, *, #8029, .F. ) ;
#5744=DIRECTION ( 'NONE',  ( -0.9685006480810791629, 2.034481705827060032E-16, -0.2490110332224850231 ) ) ;
#5757=CARTESIAN_POINT ( 'NONE',  ( 28.87608719841374949, 30.55334249999999940, -15.73691681567849976 ) ) ;
#5764=DIRECTION ( 'NONE',  ( -0.2490110332224850509, 0.000000000000000000, 0.9685006480810792739 ) ) ;
#5791=CARTESIAN_POINT ( 'NONE',  ( 28.87608719841374949, 39.28205249999999893, -15.73691681567849976 ) ) ;
#5796=VERTEX_POINT ( 'NONE', #19875 ) ;
#5817=EDGE_CURVE ( 'NONE', #2994, #6208, #14939, .T. ) ;
#5820=CARTESIAN_POINT ( 'NONE',  ( 19.51141091471011180, 2.770822500000000854, -1.622220754415315547 ) ) ;
#5840=EDGE_LOOP ( 'NONE', ( #13771, #19288, #5462, #66 ) ) ;
#5842=CARTESIAN_POINT ( 'NONE',  ( 29.64606458365116737, -6.752907499999998286, -15.53894806404596096 ) ) ;
#5845=ORIENTED_EDGE ( 'NONE', *, *, #6825, .F. ) ;
#5848=DIRECTION ( 'NONE',  ( 0.000000000000000000, -1.000000000000000000, 0.000000000000000000 ) ) ;
#5851=EDGE_LOOP ( 'NONE', ( #14339, #10537, #9365, #3438, #9246, #20222 ) ) ;
#5856=ORIENTED_EDGE ( 'NONE', *, *, #17317, .T. ) ;
#5858=CARTESIAN_POINT ( 'NONE',  ( 29.64606458365116737, -7.547927499999999235, -15.53894806404596096 ) ) ;
#5899=EDGE_CURVE ( 'NONE', #6208, #14041, #1484, .T. ) ;
#5901=VECTOR ( 'NONE', #16551, 1000.000000000000000 ) ;
#5927=VERTEX_POINT ( 'NONE', #8371 ) ;
#5931=CARTESIAN_POINT ( 'NONE',  ( 14.33584040382675262, 24.59767750000000319, -46.84351661546690337 ) ) ;
#5935=ORIENTED_EDGE ( 'NONE', *, *, #3642, .T. ) ;
#5949=CARTESIAN_POINT ( 'NONE',  ( 29.64606458365116737, -7.547927499999999235, -15.53894806404596096 ) ) ;
#5956=LINE ( 'NONE', #9163, #15251 ) ;
#5960=DIRECTION ( 'NONE',  ( 0.000000000000000000, 1.000000000000000000, 0.000000000000000000 ) ) ;
#5974=ADVANCED_FACE ( 'NONE', ( #17217 ), #13594, .F. ) ;
#5995=ADVANCED_FACE ( 'NONE', ( #8696 ), #15475, .F. ) ;
#5998=CIRCLE ( 'NONE', #11659, 1.587500000000001688 ) ;
#6003=LINE ( 'NONE', #9651, #13198 ) ;
#6024=FACE_OUTER_BOUND ( 'NONE', #1194, .T. ) ;
#6056=CIRCLE ( 'NONE', #21244, 0.7950200000000003930 ) ;
#6066=CARTESIAN_POINT ( 'NONE',  ( 2.492193568723835462, 5.548947500000001476, -24.56873394466936134 ) ) ;
#6071=CARTESIAN_POINT ( 'NONE',  ( 8.505511374756364873, -3.966527499999997097, -20.97439202360551747 ) ) ;
#6072=CARTESIAN_POINT ( 'NONE',  ( 4.766637503084914407, -6.752907499999998286, -3.239749061574506150 ) ) ;
#6074=VERTEX_POINT ( 'NONE', #4719 ) ;
#6076=CARTESIAN_POINT ( 'NONE',  ( 14.13556150701963254, -0.7997824999999986195, -46.89501028779991287 ) ) ;
#6089=CARTESIAN_POINT ( 'NONE',  ( 12.62386444219163373, 19.43957250000000059, -17.86660850434754266 ) ) ;
#6108=CIRCLE ( 'NONE', #9990, 1.983740000000001391 ) ;
#6114=VECTOR ( 'NONE', #19144, 1000.000000000000000 ) ;
#6119=DIRECTION ( 'NONE',  ( 0.9488823340533348860, -0.2002559181062069926, 0.2439669719141008553 ) ) ;
#6120=DIRECTION ( 'NONE',  ( 0.2490110332224850509, 0.000000000000000000, -0.9685006480810792739 ) ) ;
#6123=VERTEX_POINT ( 'NONE', #16546 ) ;
#6137=CARTESIAN_POINT ( 'NONE',  ( 16.85197508397059707, 13.08957250000000094, -16.77951971243562923 ) ) ;
#6152=EDGE_LOOP ( 'NONE', ( #5506, #18102, #17963, #9276 ) ) ;
#6158=EDGE_CURVE ( 'NONE', #8937, #11827, #8240, .T. ) ;
#6167=VERTEX_POINT ( 'NONE', #21619 ) ;
#6171=AXIS2_PLACEMENT_3D ( 'NONE', #5624, #7397, #20874 ) ;
#6178=CARTESIAN_POINT ( 'NONE',  ( 28.87608719841374949, 40.07707250000000698, -15.73691681567849976 ) ) ;
#6179=DIRECTION ( 'NONE',  ( 0.9685006480810791629, 0.000000000000000000, 0.2490110332224850231 ) ) ;
#6184=ORIENTED_EDGE ( 'NONE', *, *, #21665, .F. ) ;
#6199=VERTEX_POINT ( 'NONE', #9883 ) ;
#6202=DIRECTION ( 'NONE',  ( 0.000000000000000000, -1.000000000000000000, 0.000000000000000000 ) ) ;
#6208=VERTEX_POINT ( 'NONE', #3275 ) ;
#6209=LINE ( 'NONE', #9311, #11351 ) ;
#6212=FACE_OUTER_BOUND ( 'NONE', #5840, .T. ) ;
#6215=CARTESIAN_POINT ( 'NONE',  ( 23.49608546833631451, 28.96330250000000461, -17.12016812500874252 ) ) ;
#6223=DIRECTION ( 'NONE',  ( -0.8609107660235849613, 0.000000000000000000, 0.5087559856598092844 ) ) ;
#6257=DIRECTION ( 'NONE',  ( 0.9685006480810793850, 0.000000000000000000, 0.2490110332224849121 ) ) ;
#6272=LINE ( 'NONE', #4416, #12078 ) ;
#6273=CARTESIAN_POINT ( 'NONE',  ( 1.998220421679061776, -1.515722362770699494, -22.64748046904500356 ) ) ;
#6283=EDGE_LOOP ( 'NONE', ( #16160, #7434, #12663, #4123 ) ) ;
#6289=ORIENTED_EDGE ( 'NONE', *, *, #21665, .T. ) ;
#6292=VECTOR ( 'NONE', #6349, 1000.000000000000114 ) ;
#6315=ORIENTED_EDGE ( 'NONE', *, *, #1935, .F. ) ;
#6349=DIRECTION ( 'NONE',  ( -0.8609107660235849613, 0.000000000000000000, 0.5087559856598092844 ) ) ;
#6351=CIRCLE ( 'NONE', #21878, 0.7950200000000005041 ) ;
#6353=VECTOR ( 'NONE', #2772, 1000.000000000000114 ) ;
#6354=EDGE_CURVE ( 'NONE', #490, #17754, #1804, .T. ) ;
#6360=AXIS2_PLACEMENT_3D ( 'NONE', #1884, #7309, #8631 ) ;
#6366=VECTOR ( 'NONE', #1282, 1000.000000000000114 ) ;
#6377=VECTOR ( 'NONE', #13383, 1000.000000000000114 ) ;
#6381=EDGE_CURVE ( 'NONE', #15355, #21755, #4242, .T. ) ;
#6420=DIRECTION ( 'NONE',  ( -0.8609107660235850723, 0.000000000000000000, 0.5087559856598092844 ) ) ;
#6426=AXIS2_PLACEMENT_3D ( 'NONE', #20406, #15706, #7175 ) ;
#6435=AXIS2_PLACEMENT_3D ( 'NONE', #15941, #14176, #12507 ) ;
#6447=LINE ( 'NONE', #13102, #19530 ) ;
#6461=EDGE_CURVE ( 'NONE', #2495, #9790, #9176, .T. ) ;
#6472=VECTOR ( 'NONE', #20341, 1000.000000000000114 ) ;
#6491=LINE ( 'NONE', #18214, #4962 ) ;
#6498=ORIENTED_EDGE ( 'NONE', *, *, #16291, .T. ) ;
#6521=EDGE_CURVE ( 'NONE', #1632, #7768, #3923, .T. ) ;
#6524=ORIENTED_EDGE ( 'NONE', *, *, #13177, .F. ) ;
#6528=AXIS2_PLACEMENT_3D ( 'NONE', #15822, #21093, #4084 ) ;
#6536=ORIENTED_EDGE ( 'NONE', *, *, #21577, .T. ) ;
#6544=EDGE_CURVE ( 'NONE', #13842, #11503, #7664, .T. ) ;
#6548=DIRECTION ( 'NONE',  ( 0.000000000000000000, 1.000000000000000000, 0.000000000000000000 ) ) ;
#6565=CARTESIAN_POINT ( 'NONE',  ( 8.781357490942916399, 40.07707250000000698, -18.85455479843708559 ) ) ;
#6581=B_SPLINE_CURVE_WITH_KNOTS ( 'NONE', 3,
 ( #18529, #8901, #20276, #20380 ),
 .UNSPECIFIED., .F., .F.,
 ( 4, 4 ),
 ( 0.000000000000000000, 1.000000000000000000 ),
 .UNSPECIFIED. ) ;
#6619=( BOUNDED_CURVE ( )  B_SPLINE_CURVE ( 3, ( #12551, #20935, #594, #15659 ),
 .UNSPECIFIED., .F., .F. ) 
 B_SPLINE_CURVE_WITH_KNOTS ( ( 4, 4 ),
 ( 4.712388980401398086, 6.283185307179586232 ),
 .UNSPECIFIED. ) 
 CURVE ( )  GEOMETRIC_REPRESENTATION_ITEM ( )  RATIONAL_B_SPLINE_CURVE ( ( 1.000000000000000000, 0.8047378541283031206, 0.8047378541283031206, 1.000000000000000000 ) ) 
 REPRESENTATION_ITEM ( '' )  );
#6620=ORIENTED_EDGE ( 'NONE', *, *, #203, .T. ) ;
#6625=DIRECTION ( 'NONE',  ( 0.000000000000000000, -1.000000000000000000, 0.000000000000000000 ) ) ;
#6636=LINE ( 'NONE', #3340, #16328 ) ;
#6639=VECTOR ( 'NONE', #3831, 1000.000000000000114 ) ;
#6665=ORIENTED_EDGE ( 'NONE', *, *, #3642, .F. ) ;
#6671=ORIENTED_EDGE ( 'NONE', *, *, #6354, .F. ) ;
#6674=CARTESIAN_POINT ( 'NONE',  ( -7.782183222552548685, -1.594802499995993328, -34.19446947474821741 ) ) ;
#6711=ORIENTED_EDGE ( 'NONE', *, *, #7383, .F. ) ;
#6721=LINE ( 'NONE', #18548, #5617 ) ;
#6722=ORIENTED_EDGE ( 'NONE', *, *, #6521, .T. ) ;
#6754=VECTOR ( 'NONE', #21840, 1000.000000000000114 ) ;
#6761=CARTESIAN_POINT ( 'NONE',  ( 1.670997140563193373, -1.594802499999999013, -22.76294857149378714 ) ) ;
#6790=VECTOR ( 'NONE', #20769, 1000.000000000000114 ) ;
#6791=DIRECTION ( 'NONE',  ( 0.000000000000000000, -1.000000000000000000, 0.000000000000000000 ) ) ;
#6792=ORIENTED_EDGE ( 'NONE', *, *, #16578, .F. ) ;
#6825=EDGE_CURVE ( 'NONE', #14729, #18381, #7084, .T. ) ;
#6845=ORIENTED_EDGE ( 'NONE', *, *, #6158, .T. ) ;
#6859=VECTOR ( 'NONE', #3269, 1000.000000000000114 ) ;
#6882=ADVANCED_FACE ( 'NONE', ( #3887 ), #565, .T. ) ;
#6893=EDGE_LOOP ( 'NONE', ( #21095, #10979, #1809, #457 ) ) ;
#6896=DIRECTION ( 'NONE',  ( 0.2490110332224850231, 0.000000000000000000, -0.9685006480810791629 ) ) ;
#6906=CIRCLE ( 'NONE', #14337, 0.7950200000000003930 ) ;
#6910=ORIENTED_EDGE ( 'NONE', *, *, #18562, .T. ) ;
#6914=DIRECTION ( 'NONE',  ( -0.9685006480810792739, 0.000000000000000000, -0.2490110332224850509 ) ) ;
#6933=ORIENTED_EDGE ( 'NONE', *, *, #12897, .F. ) ;
#6934=CARTESIAN_POINT ( 'NONE',  ( 23.77193158452286781, 2.770822500000000854, -15.00033089984030887 ) ) ;
#6935=DIRECTION ( 'NONE',  ( 0.000000000000000000, -1.000000000000000000, 0.000000000000000000 ) ) ;
#6951=ORIENTED_EDGE ( 'NONE', *, *, #14688, .F. ) ;
#6967=ORIENTED_EDGE ( 'NONE', *, *, #19213, .F. ) ;
#6972=LINE ( 'NONE', #3780, #8048 ) ;
#6981=CARTESIAN_POINT ( 'NONE',  ( -2.234700160307072192, 26.98019749999999917, -24.80708529208898483 ) ) ;
#6982=DIRECTION ( 'NONE',  ( 0.000000000000000000, 1.000000000000000000, 0.000000000000000000 ) ) ;
#6984=PLANE ( 'NONE',  #20659 ) ;
#6987=AXIS2_PLACEMENT_3D ( 'NONE', #4212, #5764, #15626 ) ;
#7020=DIRECTION ( 'NONE',  ( 0.9685006480810791629, -4.068963411654120556E-16, 0.2490110332224850231 ) ) ;
#7023=ORIENTED_EDGE ( 'NONE', *, *, #4693, .T. ) ;
#7041=DIRECTION ( 'NONE',  ( 0.000000000000000000, -1.000000000000000000, 0.000000000000000000 ) ) ;
#7044=AXIS2_PLACEMENT_3D ( 'NONE', #435, #5508, #7186 ) ;
#7056=ADVANCED_FACE ( 'NONE', ( #9394 ), #12726, .T. ) ;
#7059=EDGE_CURVE ( 'NONE', #1295, #4521, #15583, .T. ) ;
#7084=LINE ( 'NONE', #12066, #4602 ) ;
#7102=CARTESIAN_POINT ( 'NONE',  ( 7.735533989518945219, 6.343967500000000648, -21.17236077523805449 ) ) ;
#7105=ADVANCED_FACE ( 'NONE', ( #892 ), #21218, .T. ) ;
#7106=AXIS2_PLACEMENT_3D ( 'NONE', #5791, #12550, #18169 ) ;
#7123=VECTOR ( 'NONE', #20657, 1000.000000000000000 ) ;
#7159=AXIS2_PLACEMENT_3D ( 'NONE', #3181, #20391, #8584 ) ;
#7169=DIRECTION ( 'NONE',  ( -0.5087559856598092844, 0.000000000000000000, -0.8609107660235849613 ) ) ;
#7175=DIRECTION ( 'NONE',  ( 0.9685006480810792739, 0.000000000000000000, 0.2490110332224850509 ) ) ;
#7186=DIRECTION ( 'NONE',  ( 0.000000000000000000, 1.000000000000000000, 0.000000000000000000 ) ) ;
#7196=ORIENTED_EDGE ( 'NONE', *, *, #16138, .T. ) ;
#7229=DIRECTION ( 'NONE',  ( 0.2490110332224850509, 0.000000000000000000, -0.9685006480810792739 ) ) ;
#7235=CARTESIAN_POINT ( 'NONE',  ( -2.845411283647486300, -0.7997824999999986195, -5.196881601526627925 ) ) ;
#7245=EDGE_LOOP ( 'NONE', ( #2192, #15565, #2815, #7023, #9253, #6289, #13673, #20826 ) ) ;
#7255=AXIS2_PLACEMENT_3D ( 'NONE', #9377, #1200, #19553 ) ;
#7264=DIRECTION ( 'NONE',  ( 0.9685006480810792739, -0.000000000000000000, 0.2490110332224850509 ) ) ;
#7269=CARTESIAN_POINT ( 'NONE',  ( -4.728951812473551897, 2.373947500000000765, -29.02782796843600011 ) ) ;
#7274=CARTESIAN_POINT ( 'NONE',  ( 8.011380105705496746, -6.752907499999998286, -19.05252355006962617 ) ) ;
#7309=DIRECTION ( 'NONE',  ( -0.5171931484643310650, -0.000000000000000000, -0.8558687090795833452 ) ) ;
#7315=EDGE_CURVE ( 'NONE', #1762, #5667, #15153, .T. ) ;
#7321=FACE_OUTER_BOUND ( 'NONE', #9418, .T. ) ;
#7325=DIRECTION ( 'NONE',  ( 0.000000000000000000, -1.000000000000000000, 0.000000000000000000 ) ) ;
#7336=PRODUCT_CONTEXT ( 'NONE', #13863, 'mechanical' ) ;
#7339=( BOUNDED_CURVE ( )  B_SPLINE_CURVE ( 3, ( #21880, #20211, #1645, #15061 ),
 .UNSPECIFIED., .F., .T. ) 
 B_SPLINE_CURVE_WITH_KNOTS ( ( 4, 4 ),
 ( 4.712388980383330761, 6.283185307179586232 ),
 .UNSPECIFIED. ) 
 CURVE ( )  GEOMETRIC_REPRESENTATION_ITEM ( )  RATIONAL_B_SPLINE_CURVE ( ( 1.000000000000000000, 0.8047378541240446381, 0.8047378541240446381, 1.000000000000000000 ) ) 
 REPRESENTATION_ITEM ( '' )  );
#7345=DIRECTION ( 'NONE',  ( -0.8609107660235850723, 0.000000000000000000, 0.5087559856598092844 ) ) ;
#7364=ORIENTED_EDGE ( 'NONE', *, *, #5593, .T. ) ;
#7381=EDGE_CURVE ( 'NONE', #7442, #11658, #12675, .T. ) ;
#7383=EDGE_CURVE ( 'NONE', #490, #6167, #8484, .T. ) ;
#7397=DIRECTION ( 'NONE',  ( 0.2490110332224850509, 0.000000000000000000, -0.9685006480810792739 ) ) ;
#7434=ORIENTED_EDGE ( 'NONE', *, *, #11131, .F. ) ;
#7437=AXIS2_PLACEMENT_3D ( 'NONE', #19295, #10796, #13606 ) ;
#7442=VERTEX_POINT ( 'NONE', #7586 ) ;
#7444=CARTESIAN_POINT ( 'NONE',  ( 9.275488759993784527, -7.547927499999999235, -20.77642327197297689 ) ) ;
#7446=ORIENTED_EDGE ( 'NONE', *, *, #9890, .F. ) ;
#7459=EDGE_CURVE ( 'NONE', #18381, #18451, #16966, .T. ) ;
#7460=ORIENTED_EDGE ( 'NONE', *, *, #11667, .T. ) ;
#7472=DIRECTION ( 'NONE',  ( 0.000000000000000000, 1.000000000000000000, 0.000000000000000000 ) ) ;
#7481=ORIENTED_EDGE ( 'NONE', *, *, #19951, .F. ) ;
#7488=VECTOR ( 'NONE', #2438, 1000.000000000000114 ) ;
#7489=VERTEX_POINT ( 'NONE', #12038 ) ;
#7510=( GEOMETRIC_REPRESENTATION_CONTEXT ( 3 ) GLOBAL_UNCERTAINTY_ASSIGNED_CONTEXT ( ( #5688 ) ) GLOBAL_UNIT_ASSIGNED_CONTEXT ( ( #16367, #7836, #19761 ) ) REPRESENTATION_CONTEXT ( 'NONE', 'WORKASPACE' ) );
#7521=DIRECTION ( 'NONE',  ( 0.2490110332224850509, 0.000000000000000000, -0.9685006480810792739 ) ) ;
#7522=AXIS2_PLACEMENT_3D ( 'NONE', #11379, #16148, #9598 ) ;
#7526=DIRECTION ( 'NONE',  ( 0.2490110332224850509, 0.000000000000000000, -0.9685006480810792739 ) ) ;
#7537=EDGE_CURVE ( 'NONE', #2498, #18746, #9210, .T. ) ;
#7541=DIRECTION ( 'NONE',  ( 0.9685006480810792739, 0.000000000000000000, 0.2490110332224850509 ) ) ;
#7543=LINE ( 'NONE', #578, #6114 ) ;
#7554=CIRCLE ( 'NONE', #20243, 0.7950200000000005041 ) ;
#7586=CARTESIAN_POINT ( 'NONE',  ( -7.949728765565600597, 33.32892749999999893, -34.47798802950714503 ) ) ;
#7593=CARTESIAN_POINT ( 'NONE',  ( -3.037751992662818257, 28.56769750000000130, -30.02724401157551526 ) ) ;
#7601=ORIENTED_EDGE ( 'NONE', *, *, #2239, .T. ) ;
#7614=EDGE_CURVE ( 'NONE', #10018, #21869, #1048, .T. ) ;
#7621=DIRECTION ( 'NONE',  ( 0.8609107660235849613, 0.000000000000000000, -0.5087559856598092844 ) ) ;
#7623=FILL_AREA_STYLE ('',( #11052 ) ) ;
#7630=VERTEX_POINT ( 'NONE', #21608 ) ;
#7652=ORIENTED_EDGE ( 'NONE', *, *, #11927, .T. ) ;
#7660=EDGE_CURVE ( 'NONE', #14970, #14236, #12794, .T. ) ;
#7663=ORIENTED_EDGE ( 'NONE', *, *, #8093, .T. ) ;
#7664=LINE ( 'NONE', #6215, #21222 ) ;
#7682=EDGE_CURVE ( 'NONE', #12681, #8349, #3228, .T. ) ;
#7687=DIRECTION ( 'NONE',  ( 0.9685006480810792739, 0.000000000000000000, 0.2490110332224850509 ) ) ;
#7693=AXIS2_PLACEMENT_3D ( 'NONE', #16492, #16711, #1438 ) ;
#7700=EDGE_LOOP ( 'NONE', ( #1840, #14772, #12923, #17093 ) ) ;
#7732=EDGE_CURVE ( 'NONE', #6199, #21155, #9559, .T. ) ;
#7766=CARTESIAN_POINT ( 'NONE',  ( 8.011380105705496746, 34.12394749999999988, -19.05252355006962617 ) ) ;
#7768=VERTEX_POINT ( 'NONE', #16452 ) ;
#7775=CARTESIAN_POINT ( 'NONE',  ( 23.00195419928544638, 3.565842500000000914, -15.19829965147284945 ) ) ;
#7780=LINE ( 'NONE', #17326, #9719 ) ;
#7782=DIRECTION ( 'NONE',  ( -0.5087559856598092844, 0.000000000000000000, -0.8609107660235849613 ) ) ;
#7807=VERTEX_POINT ( 'NONE', #8248 ) ;
#7825=CARTESIAN_POINT ( 'NONE',  ( -0.8970842057359728061, 5.548947500000001476, -22.54358764576276286 ) ) ;
#7826=CARTESIAN_POINT ( 'NONE',  ( 0.2641497867371597752, 5.548947500000001476, -24.43980549416641068 ) ) ;
#7834=DIRECTION ( 'NONE',  ( 0.2490110332224850231, 0.000000000000000000, -0.9685006480810791629 ) ) ;
#7836=( NAMED_UNIT ( * ) PLANE_ANGLE_UNIT ( ) SI_UNIT ( $, .RADIAN. ) );
#7837=FACE_OUTER_BOUND ( 'NONE', #13710, .T. ) ;
#7842=DIRECTION ( 'NONE',  ( 0.2490110332224850509, 0.000000000000000000, -0.9685006480810792739 ) ) ;
#7851=VECTOR ( 'NONE', #1473, 1000.000000000000000 ) ;
#7856=DIRECTION ( 'NONE',  ( -0.2490110332224850509, 0.000000000000000000, 0.9685006480810792739 ) ) ;
#7860=ORIENTED_EDGE ( 'NONE', *, *, #13177, .T. ) ;
#7862=CARTESIAN_POINT ( 'NONE',  ( -1.351150467732365579, 26.98019749999999917, -27.17319717629097653 ) ) ;
#7881=VECTOR ( 'NONE', #17492, 1000.000000000000000 ) ;
#7886=DIRECTION ( 'NONE',  ( -0.9685006480810792739, 0.000000000000000000, -0.2490110332224850231 ) ) ;
#7890=CYLINDRICAL_SURFACE ( 'NONE', #20535, 0.7950200000000005041 ) ;
#7903=DIRECTION ( 'NONE',  ( -0.8609107660235848503, 0.000000000000000000, 0.5087559856598096175 ) ) ;
#7939=VECTOR ( 'NONE', #13293, 1000.000000000000114 ) ;
#7958=CIRCLE ( 'NONE', #183, 0.7950200000000000600 ) ;
#7995=EDGE_CURVE ( 'NONE', #10315, #21656, #20689, .T. ) ;
#7996=FACE_OUTER_BOUND ( 'NONE', #17675, .T. ) ;
#8000=CARTESIAN_POINT ( 'NONE',  ( -4.728951812473551897, 28.56769750000000130, -29.02782796843600011 ) ) ;
#8001=ORIENTED_EDGE ( 'NONE', *, *, #4912, .F. ) ;
#8029=EDGE_CURVE ( 'NONE', #10927, #10511, #15238, .T. ) ;
#8034=ORIENTED_EDGE ( 'NONE', *, *, #5527, .T. ) ;
#8048=VECTOR ( 'NONE', #4001, 1000.000000000000114 ) ;
#8076=CARTESIAN_POINT ( 'NONE',  ( 5.430521817098937554, -1.594802499999999013, -21.76500205408690647 ) ) ;
#8092=CARTESIAN_POINT ( 'NONE',  ( 1.445847263472733291, 34.12394749999999988, -6.267054683493481271 ) ) ;
#8093=EDGE_CURVE ( 'NONE', #513, #18859, #18357, .T. ) ;
#8099=ORIENTED_EDGE ( 'NONE', *, *, #11131, .T. ) ;
#8105=DIRECTION ( 'NONE',  ( 0.2490110332224850509, 0.000000000000000000, -0.9685006480810792739 ) ) ;
#8137=ORIENTED_EDGE ( 'NONE', *, *, #5399, .T. ) ;
#8149=EDGE_CURVE ( 'NONE', #15355, #7442, #6636, .T. ) ;
#8161=DIRECTION ( 'NONE',  ( 0.000000000000000000, 1.000000000000000000, 0.000000000000000000 ) ) ;
#8168=VECTOR ( 'NONE', #2898, 1000.000000000000000 ) ;
#8176=EDGE_CURVE ( 'NONE', #11803, #2298, #15974, .T. ) ;
#8182=PLANE ( 'NONE',  #19566 ) ;
#8200=VECTOR ( 'NONE', #1093, 1000.000000000000114 ) ;
#8229=( LENGTH_UNIT ( ) NAMED_UNIT ( * ) SI_UNIT ( .MILLI., .METRE. ) );
#8237=VERTEX_POINT ( 'NONE', #10621 ) ;
#8240=LINE ( 'NONE', #1494, #12044 ) ;
#8248=CARTESIAN_POINT ( 'NONE',  ( 29.64606458365116737, -1.985327499999998357, -15.53894806404596096 ) ) ;
#8253=CARTESIAN_POINT ( 'NONE',  ( 8.781357490942916399, -7.547927499999999235, -18.85455479843708559 ) ) ;
#8293=ORIENTED_EDGE ( 'NONE', *, *, #21610, .T. ) ;
#8297=LINE ( 'NONE', #16814, #5010 ) ;
#8299=AXIS2_PLACEMENT_3D ( 'NONE', #9592, #16361, #21420 ) ;
#8320=CARTESIAN_POINT ( 'NONE',  ( 7.735533989518945219, 5.548947500000001476, -21.17236077523805449 ) ) ;
#8324=CARTESIAN_POINT ( 'NONE',  ( 23.49608546833631451, 28.96330250000000461, -17.12016812500874252 ) ) ;
#8331=CARTESIAN_POINT ( 'NONE',  ( 28.38195592936287781, 30.55334249999999940, -13.81504834214261024 ) ) ;
#8346=EDGE_CURVE ( 'NONE', #9048, #21748, #5956, .T. ) ;
#8347=LINE ( 'NONE', #18405, #16172 ) ;
#8349=VERTEX_POINT ( 'NONE', #12844 ) ;
#8352=DIRECTION ( 'NONE',  ( 0.9685006480810790519, 0.000000000000000000, 0.2490110332224857170 ) ) ;
#8371=CARTESIAN_POINT ( 'NONE',  ( 29.15193331460030279, 30.55334249999999940, -13.61707959051006966 ) ) ;
#8385=CARTESIAN_POINT ( 'NONE',  ( -1.427050033073577806, 5.548947500000001476, -23.44038945102687066 ) ) ;
#8386=DIRECTION ( 'NONE',  ( -0.2490110332224849676, 0.000000000000000000, 0.9685006480810792739 ) ) ;
#8400=VECTOR ( 'NONE', #12621, 1000.000000000000000 ) ;
#8452=VERTEX_POINT ( 'NONE', #9390 ) ;
#8458=DIRECTION ( 'NONE',  ( 0.5087559856598092844, 0.000000000000000000, 0.8609107660235849613 ) ) ;
#8463=ADVANCED_FACE ( 'NONE', ( #14497 ), #12955, .T. ) ;
#8484=CIRCLE ( 'NONE', #20838, 3.970020000000002991 ) ;
#8520=EDGE_CURVE ( 'NONE', #14184, #8937, #6056, .T. ) ;
#8534=CIRCLE ( 'NONE', #14575, 3.174999999999998490 ) ;
#8537=EDGE_CURVE ( 'NONE', #21183, #16767, #2175, .T. ) ;
#8541=LINE ( 'NONE', #5442, #17618 ) ;
#8549=EDGE_CURVE ( 'NONE', #21755, #17754, #19236, .T. ) ;
#8562=ORIENTED_EDGE ( 'NONE', *, *, #272, .T. ) ;
#8567=ORIENTED_EDGE ( 'NONE', *, *, #10696, .T. ) ;
#8584=DIRECTION ( 'NONE',  ( 0.9685006480810793850, 0.000000000000000000, 0.2490110332224846901 ) ) ;
#8618=VECTOR ( 'NONE', #19166, 1000.000000000000227 ) ;
#8620=DIRECTION ( 'NONE',  ( 0.5087559856598088404, 0.000000000000000000, 0.8609107660235851833 ) ) ;
#8621=CARTESIAN_POINT ( 'NONE',  ( 1.173720826352361080, 34.12394749999999988, -20.82884779549221577 ) ) ;
#8631=DIRECTION ( 'NONE',  ( 0.000000000000000000, -1.000000000000000000, 0.000000000000000000 ) ) ;
#8639=AXIS2_PLACEMENT_3D ( 'NONE', #18664, #3427, #1646 ) ;
#8693=ADVANCED_FACE ( 'NONE', ( #308 ), #15585, .F. ) ;
#8696=FACE_OUTER_BOUND ( 'NONE', #14178, .T. ) ;
#8699=ORIENTED_EDGE ( 'NONE', *, *, #3894, .F. ) ;
#8708=CARTESIAN_POINT ( 'NONE',  ( -3.042350287543033716, 26.98019749999999917, -26.17378113315171007 ) ) ;
#8717=CARTESIAN_POINT ( 'NONE',  ( 30.86636926788154156, 3.565842500000000914, -42.59335521360503662 ) ) ;
#8722=ORIENTED_EDGE ( 'NONE', *, *, #10148, .F. ) ;
#8726=CARTESIAN_POINT ( 'NONE',  ( 23.00195419928544638, 3.565842500000000914, -15.19829965147284945 ) ) ;
#8732=ORIENTED_EDGE ( 'NONE', *, *, #7459, .F. ) ;
#8779=LINE ( 'NONE', #18848, #3868 ) ;
#8797=VERTEX_POINT ( 'NONE', #635 ) ;
#8800=DIRECTION ( 'NONE',  ( 0.9685006480810791629, 0.000000000000000000, 0.2490110332224850231 ) ) ;
#8802=LINE ( 'NONE', #2180, #14462 ) ;
#8809=ORIENTED_EDGE ( 'NONE', *, *, #8149, .T. ) ;
#8820=AXIS2_PLACEMENT_3D ( 'NONE', #17935, #9515, #16285 ) ;
#8826=DIRECTION ( 'NONE',  ( -0.8609107660235848503, 0.000000000000000000, 0.5087559856598096175 ) ) ;
#8839=CARTESIAN_POINT ( 'NONE',  ( -1.351150467732365579, 3.961447500000001565, -27.17319717629097653 ) ) ;
#8878=CIRCLE ( 'NONE', #9587, 2.182812499999999378 ) ;
#8890=CARTESIAN_POINT ( 'NONE',  ( -3.845402119898529758, 26.98019749999999917, -31.39393985263922460 ) ) ;
#8896=ADVANCED_FACE ( 'NONE', ( #9252 ), #16031, .F. ) ;
#8898=FACE_OUTER_BOUND ( 'NONE', #10710, .T. ) ;
#8901=CARTESIAN_POINT ( 'NONE',  ( 1.776692311943213420, -1.594802499999998124, -22.71488278333245603 ) ) ;
#8904=VECTOR ( 'NONE', #18736, 1000.000000000000000 ) ;
#8909=CARTESIAN_POINT ( 'NONE',  ( -7.545238043312568088, 34.12394749999999988, -33.79351368943453338 ) ) ;
#8916=CARTESIAN_POINT ( 'NONE',  ( -0.8970842057359728061, 34.12394749999999988, -22.54358764576276286 ) ) ;
#8920=FACE_OUTER_BOUND ( 'NONE', #13783, .T. ) ;
#8935=EDGE_LOOP ( 'NONE', ( #8722, #18397, #14584, #14040 ) ) ;
#8937=VERTEX_POINT ( 'NONE', #12816 ) ;
#8948=LINE ( 'NONE', #15726, #11709 ) ;
#8963=CARTESIAN_POINT ( 'NONE',  ( 8.505511374756364873, -6.752907499999998286, -20.97439202360551747 ) ) ;
#8984=DIRECTION ( 'NONE',  ( -0.2490110332224850231, 0.000000000000000000, 0.9685006480810791629 ) ) ;
#9010=CARTESIAN_POINT ( 'NONE',  ( -0.8970842057359728061, 25.39269750000000059, -22.54358764576276286 ) ) ;
#9012=DIRECTION ( 'NONE',  ( -0.000000000000000000, 1.000000000000000000, 0.000000000000000000 ) ) ;
#9034=DIRECTION ( 'NONE',  ( -0.2490110332224850509, 0.000000000000000000, 0.9685006480810792739 ) ) ;
#9048=VERTEX_POINT ( 'NONE', #8253 ) ;
#9062=ORIENTED_EDGE ( 'NONE', *, *, #16650, .T. ) ;
#9076=DIRECTION ( 'NONE',  ( 0.000000000000000000, 1.000000000000000000, 0.000000000000000000 ) ) ;
#9083=ORIENTED_EDGE ( 'NONE', *, *, #16650, .F. ) ;
#9098=CYLINDRICAL_SURFACE ( 'NONE', #16014, 1.587500000000002132 ) ;
#9104=ORIENTED_EDGE ( 'NONE', *, *, #11086, .T. ) ;
#9110=DIRECTION ( 'NONE',  ( 0.9685006480810792739, -0.000000000000000000, 0.2490110332224850509 ) ) ;
#9159=ORIENTED_EDGE ( 'NONE', *, *, #20990, .F. ) ;
#9160=VERTEX_POINT ( 'NONE', #10128 ) ;
#9163=CARTESIAN_POINT ( 'NONE',  ( 8.781357490942916399, -7.547927499999999235, -18.85455479843708559 ) ) ;
#9176=B_SPLINE_CURVE_WITH_KNOTS ( 'NONE', 3,
 ( #5448, #12210, #2250, #3804 ),
 .UNSPECIFIED., .F., .F.,
 ( 4, 4 ),
 ( 0.000000000000000000, 1.000000000000000000 ),
 .UNSPECIFIED. ) ;
#9179=DIRECTION ( 'NONE',  ( 0.000000000000000000, -1.000000000000000000, 0.000000000000000000 ) ) ;
#9194=ADVANCED_FACE ( 'NONE', ( #510 ), #15562, .F. ) ;
#9203=CIRCLE ( 'NONE', #4269, 1.587499999999998579 ) ;
#9210=CIRCLE ( 'NONE', #399, 1.587499999999998579 ) ;
#9214=PRODUCT_DEFINITION_CONTEXT ( 'detailed design', #14579, 'design' ) ;
#9226=EDGE_CURVE ( 'NONE', #8349, #2994, #6581, .T. ) ;
#9232=CARTESIAN_POINT ( 'NONE',  ( 8.505511374756364873, 24.59767750000000319, -20.97439202360551747 ) ) ;
#9246=ORIENTED_EDGE ( 'NONE', *, *, #16267, .F. ) ;
#9252=FACE_OUTER_BOUND ( 'NONE', #21412, .T. ) ;
#9253=ORIENTED_EDGE ( 'NONE', *, *, #5899, .T. ) ;
#9266=CYLINDRICAL_SURFACE ( 'NONE', #14680, 1.983740000000001391 ) ;
#9272=LINE ( 'NONE', #879, #5368 ) ;
#9276=ORIENTED_EDGE ( 'NONE', *, *, #2078, .F. ) ;
#9277=ORIENTED_EDGE ( 'NONE', *, *, #18199, .T. ) ;
#9282=ORIENTED_EDGE ( 'NONE', *, *, #18241, .F. ) ;
#9293=DIRECTION ( 'NONE',  ( 0.8609107660235850723, 0.000000000000000000, -0.5087559856598092844 ) ) ;
#9298=LINE ( 'NONE', #9510, #21526 ) ;
#9311=CARTESIAN_POINT ( 'NONE',  ( 29.64606458365116737, 36.49567249999999774, -15.53894806404596096 ) ) ;
#9365=ORIENTED_EDGE ( 'NONE', *, *, #8537, .T. ) ;
#9377=CARTESIAN_POINT ( 'NONE',  ( 24.26606285357373594, 3.565842500000000914, -16.92219937337620195 ) ) ;
#9382=CARTESIAN_POINT ( 'NONE',  ( 13.11799571124250363, 13.08957250000000094, -19.78847697788343396 ) ) ;
#9390=CARTESIAN_POINT ( 'NONE',  ( 29.64606458365116737, -3.966527499999997097, -15.53894806404596096 ) ) ;
#9394=FACE_OUTER_BOUND ( 'NONE', #1560, .T. ) ;
#9403=DIRECTION ( 'NONE',  ( 0.000000000000000000, 1.000000000000000000, 0.000000000000000000 ) ) ;
#9416=CARTESIAN_POINT ( 'NONE',  ( 29.64606458365116737, 30.55334249999999940, -15.53894806404596096 ) ) ;
#9418=EDGE_LOOP ( 'NONE', ( #12375, #13618, #13059, #17624 ) ) ;
#9419=DIRECTION ( 'NONE',  ( 0.000000000000000000, 1.000000000000000000, 0.000000000000000000 ) ) ;
#9464=DIRECTION ( 'NONE',  ( 0.2490110332224850509, 0.000000000000000000, -0.9685006480810792739 ) ) ;
#9475=ADVANCED_FACE ( 'NONE', ( #17762 ), #20958, .F. ) ;
#9510=CARTESIAN_POINT ( 'NONE',  ( 8.011380105705496746, -1.594802499999999013, -19.05252355006962617 ) ) ;
#9513=ORIENTED_EDGE ( 'NONE', *, *, #20383, .F. ) ;
#9515=DIRECTION ( 'NONE',  ( -0.2490110332224850509, 0.000000000000000000, 0.9685006480810792739 ) ) ;
#9526=CARTESIAN_POINT ( 'NONE',  ( -6.268352501591477832, -0.7997824999999986195, -35.49402737582407497 ) ) ;
#9536=AXIS2_PLACEMENT_3D ( 'NONE', #7102, #19028, #7325 ) ;
#9539=PLANE ( 'NONE',  #12828 ) ;
#9548=CARTESIAN_POINT ( 'NONE',  ( 29.15193331460030279, 39.28205249999999893, -13.61707959051006966 ) ) ;
#9559=LINE ( 'NONE', #6137, #5325 ) ;
#9584=( BOUNDED_CURVE ( )  B_SPLINE_CURVE ( 3, ( #3058, #1281, #12502, #11346 ),
 .UNSPECIFIED., .F., .T. ) 
 B_SPLINE_CURVE_WITH_KNOTS ( ( 4, 4 ),
 ( 0.000000000000000000, 1.570796326788112873 ),
 .UNSPECIFIED. ) 
 CURVE ( )  GEOMETRIC_REPRESENTATION_ITEM ( )  RATIONAL_B_SPLINE_CURVE ( ( 1.000000000000000000, 0.8047378541259639917, 0.8047378541259639917, 1.000000000000000000 ) ) 
 REPRESENTATION_ITEM ( '' )  );
#9587=AXIS2_PLACEMENT_3D ( 'NONE', #11617, #14963, #18156 ) ;
#9591=DIRECTION ( 'NONE',  ( -0.9685006480810792739, 0.000000000000000000, -0.2490110332224850231 ) ) ;
#9592=CARTESIAN_POINT ( 'NONE',  ( 15.87579517430159193, 39.28205249999999893, -46.44757911220182223 ) ) ;
#9598=DIRECTION ( 'NONE',  ( -0.5171931484643331745, 0.000000000000000000, -0.8558687090795820129 ) ) ;
#9620=LINE ( 'NONE', #6089, #1407 ) ;
#9639=CARTESIAN_POINT ( 'NONE',  ( 9.275488759993784527, 40.07707250000000698, -20.77642327197297689 ) ) ;
#9651=CARTESIAN_POINT ( 'NONE',  ( -1.351150467732365579, 2.373947500000000765, -27.17319717629097653 ) ) ;
#9655=DIRECTION ( 'NONE',  ( 0.000000000000000000, 1.000000000000000000, 0.000000000000000000 ) ) ;
#9660=CARTESIAN_POINT ( 'NONE',  ( 23.49608546833631451, 3.565842500000000914, -17.12016812500874252 ) ) ;
#9668=CARTESIAN_POINT ( 'NONE',  ( -3.037751992662818257, 28.56769750000000130, -30.02724401157551526 ) ) ;
#9676=ORIENTED_EDGE ( 'NONE', *, *, #3726, .F. ) ;
#9692=ORIENTED_EDGE ( 'NONE', *, *, #17786, .F. ) ;
#9710=SURFACE_STYLE_FILL_AREA ( #7623 ) ;
#9713=EDGE_LOOP ( 'NONE', ( #5856, #16788, #2296, #12913 ) ) ;
#9719=VECTOR ( 'NONE', #14546, 1000.000000000000114 ) ;
#9722=FACE_OUTER_BOUND ( 'NONE', #9713, .T. ) ;
#9727=DIRECTION ( 'NONE',  ( 0.000000000000000000, 1.000000000000000000, 0.000000000000000000 ) ) ;
#9734=LINE ( 'NONE', #20105, #4999 ) ;
#9753=CARTESIAN_POINT ( 'NONE',  ( 28.38195592936287781, 39.28205249999999893, -13.81504834214261024 ) ) ;
#9774=ORIENTED_EDGE ( 'NONE', *, *, #9226, .F. ) ;
#9790=VERTEX_POINT ( 'NONE', #18824 ) ;
#9826=CARTESIAN_POINT ( 'NONE',  ( 1.532169971477637782, -1.500984687155947128, -20.71839214105750315 ) ) ;
#9847=LINE ( 'NONE', #6761, #12894 ) ;
#9852=DIRECTION ( 'NONE',  ( 0.000000000000000000, 1.000000000000000000, 0.000000000000000000 ) ) ;
#9857=DIRECTION ( 'NONE',  ( 0.000000000000000000, 1.000000000000000000, 0.000000000000000000 ) ) ;
#9875=VECTOR ( 'NONE', #2569, 1000.000000000000000 ) ;
#9883=CARTESIAN_POINT ( 'NONE',  ( 16.85197508397059707, 13.08957250000000094, -16.77951971243562923 ) ) ;
#9890=EDGE_CURVE ( 'NONE', #9790, #17754, #14059, .T. ) ;
#9904=VECTOR ( 'NONE', #839, 1000.000000000000227 ) ;
#9924=LINE ( 'NONE', #18643, #2558 ) ;
#9927=ORIENTED_EDGE ( 'NONE', *, *, #7682, .F. ) ;
#9959=AXIS2_PLACEMENT_3D ( 'NONE', #16998, #300, #7041 ) ;
#9972=AXIS2_PLACEMENT_3D ( 'NONE', #15417, #244, #6982 ) ;
#9990=AXIS2_PLACEMENT_3D ( 'NONE', #10963, #15851, #12531 ) ;
#9993=DIRECTION ( 'NONE',  ( 0.000000000000000000, -1.000000000000000000, 0.000000000000000000 ) ) ;
#10005=ORIENTED_EDGE ( 'NONE', *, *, #7059, .T. ) ;
#10018=VERTEX_POINT ( 'NONE', #18892 ) ;
#10025=VECTOR ( 'NONE', #5744, 1000.000000000000114 ) ;
#10068=EDGE_LOOP ( 'NONE', ( #6910, #19538, #3152, #3390 ) ) ;
#10081=DIRECTION ( 'NONE',  ( -0.2490110332224850231, 0.000000000000000000, 0.9685006480810791629 ) ) ;
#10087=DIRECTION ( 'NONE',  ( -0.2490110332224850231, 0.000000000000000000, 0.9685006480810791629 ) ) ;
#10093=ORIENTED_EDGE ( 'NONE', *, *, #13193, .T. ) ;
#10097=EDGE_CURVE ( 'NONE', #20863, #13842, #12168, .T. ) ;
#10108=ORIENTED_EDGE ( 'NONE', *, *, #19385, .F. ) ;
#10118=ORIENTED_EDGE ( 'NONE', *, *, #7614, .T. ) ;
#10128=CARTESIAN_POINT ( 'NONE',  ( 28.87608719841374949, 2.770822500000000854, -15.73691681567849976 ) ) ;
#10132=AXIS2_PLACEMENT_3D ( 'NONE', #1952, #10581, #19083 ) ;
#10148=EDGE_CURVE ( 'NONE', #11658, #8237, #9584, .T. ) ;
#10151=CARTESIAN_POINT ( 'NONE',  ( 0.7843704457339527591, -1.594802499999999013, -23.55949434567611078 ) ) ;
#10153=ORIENTED_EDGE ( 'NONE', *, *, #5282, .T. ) ;
#10161=DIRECTION ( 'NONE',  ( 0.000000000000000000, -1.000000000000000000, 0.000000000000000000 ) ) ;
#10195=ORIENTED_EDGE ( 'NONE', *, *, #20904, .F. ) ;
#10226=EDGE_LOOP ( 'NONE', ( #21507, #18392, #19848, #10005 ) ) ;
#10227=CARTESIAN_POINT ( 'NONE',  ( 28.87608719841374949, 2.770822500000000854, -15.73691681567849976 ) ) ;
#10242=VECTOR ( 'NONE', #3567, 1000.000000000000114 ) ;
#10245=LINE ( 'NONE', #10364, #2663 ) ;
#10268=CARTESIAN_POINT ( 'NONE',  ( 1.169308704210513694, -0.7997824999999986195, -20.81168733838920915 ) ) ;
#10280=VERTEX_POINT ( 'NONE', #16126 ) ;
#10291=CARTESIAN_POINT ( 'NONE',  ( 2.520748753591570690, 102.1610225000000014, -24.56335908395234924 ) ) ;
#10306=AXIS2_PLACEMENT_3D ( 'NONE', #17696, #19663, #4530 ) ;
#10311=CARTESIAN_POINT ( 'NONE',  ( 16.85197508397059707, 19.43957250000000059, -16.77951971243562923 ) ) ;
#10315=VERTEX_POINT ( 'NONE', #17781 ) ;
#10364=CARTESIAN_POINT ( 'NONE',  ( 12.62386444219163373, 13.08957250000000094, -17.86660850434754266 ) ) ;
#10375=ORIENTED_EDGE ( 'NONE', *, *, #3726, .T. ) ;
#10388=ORIENTED_EDGE ( 'NONE', *, *, #992, .T. ) ;
#10390=LINE ( 'NONE', #647, #10025 ) ;
#10413=DIRECTION ( 'NONE',  ( 0.000000000000000000, -1.000000000000000000, 0.000000000000000000 ) ) ;
#10453=EDGE_LOOP ( 'NONE', ( #5935, #10594, #16798, #16136 ) ) ;
#10457=LINE ( 'NONE', #508, #14950 ) ;
#10458=EDGE_CURVE ( 'NONE', #5796, #18904, #5584, .T. ) ;
#10467=CARTESIAN_POINT ( 'NONE',  ( 12.62386444219163373, 19.43957250000000059, -17.86660850434754266 ) ) ;
#10468=ADVANCED_FACE ( 'NONE', ( #20330 ), #3445, .T. ) ;
#10493=EDGE_CURVE ( 'NONE', #12681, #6123, #17155, .T. ) ;
#10503=CYLINDRICAL_SURFACE ( 'NONE', #16651, 0.7950199999999971734 ) ;
#10511=VERTEX_POINT ( 'NONE', #15410 ) ;
#10523=EDGE_CURVE ( 'NONE', #13662, #1981, #6972, .T. ) ;
#10537=ORIENTED_EDGE ( 'NONE', *, *, #11086, .F. ) ;
#10548=ADVANCED_FACE ( 'NONE', ( #17489, #2223 ), #4106, .T. ) ;
#10567=VECTOR ( 'NONE', #13142, 1000.000000000000114 ) ;
#10573=DIRECTION ( 'NONE',  ( 0.000000000000000000, -1.000000000000000000, 0.000000000000000000 ) ) ;
#10577=EDGE_CURVE ( 'NONE', #18381, #21183, #1785, .T. ) ;
#10581=DIRECTION ( 'NONE',  ( 0.2490110332224850509, 0.000000000000000000, -0.9685006480810792739 ) ) ;
#10594=ORIENTED_EDGE ( 'NONE', *, *, #20990, .T. ) ;
#10609=LINE ( 'NONE', #19324, #13252 ) ;
#10613=ORIENTED_EDGE ( 'NONE', *, *, #9226, .T. ) ;
#10620=AXIS2_PLACEMENT_3D ( 'NONE', #10682, #6914, #13677 ) ;
#10621=CARTESIAN_POINT ( 'NONE',  ( -5.863861779363051419, 34.12394749999999988, -34.80955303575778714 ) ) ;
#10628=CARTESIAN_POINT ( 'NONE',  ( 1.890011456818353031, 34.09881183566065488, -22.67530205718465908 ) ) ;
#10647=VECTOR ( 'NONE', #11221, 1000.000000000000114 ) ;
#10651=DIRECTION ( 'NONE',  ( 0.9685006480810792739, 0.000000000000000000, 0.2490110332224853007 ) ) ;
#10668=CYLINDRICAL_SURFACE ( 'NONE', #14951, 1.587499999999999911 ) ;
#10669=AXIS2_PLACEMENT_3D ( 'NONE', #5263, #19086, #6935 ) ;
#10682=CARTESIAN_POINT ( 'NONE',  ( 9.133321157616299146, 13.08957250000000094, -4.290529607290007874 ) ) ;
#10683=DIRECTION ( 'NONE',  ( -0.9488823340533351081, -0.2002559181062071036, -0.2439669719140995230 ) ) ;
#10687=EDGE_CURVE ( 'NONE', #12517, #11596, #14076, .T. ) ;
#10696=EDGE_CURVE ( 'NONE', #19764, #9048, #17943, .T. ) ;
#10700=ORIENTED_EDGE ( 'NONE', *, *, #20682, .T. ) ;
#10707=ORIENTED_EDGE ( 'NONE', *, *, #20673, .F. ) ;
#10710=EDGE_LOOP ( 'NONE', ( #11161, #11707, #13605, #18213, #21538, #15054 ) ) ;
#10722=VECTOR ( 'NONE', #16514, 1000.000000000000000 ) ;
#10731=ADVANCED_FACE ( 'NONE', ( #9722 ), #16486, .F. ) ;
#10743=CARTESIAN_POINT ( 'NONE',  ( 1.998220421679061776, 34.04486736277070236, -22.64748046904500356 ) ) ;
#10747=CARTESIAN_POINT ( 'NONE',  ( 1.532169971477637782, 5.548947500000001476, -20.71839214105750315 ) ) ;
#10751=CARTESIAN_POINT ( 'NONE',  ( -3.845402119898529758, 28.56769750000000130, -31.39393985263922460 ) ) ;
#10763=CARTESIAN_POINT ( 'NONE',  ( 29.64606458365116737, 1.975802500000001904, -15.53894806404596096 ) ) ;
#10774=CIRCLE ( 'NONE', #16080, 0.7950200000000003930 ) ;
#10790=FACE_OUTER_BOUND ( 'NONE', #19770, .T. ) ;
#10796=DIRECTION ( 'NONE',  ( 0.2490110332224850509, 0.000000000000000000, -0.9685006480810792739 ) ) ;
#10816=EDGE_LOOP ( 'NONE', ( #18524, #16629, #18554, #20193, #2765, #7860 ) ) ;
#10832=DIRECTION ( 'NONE',  ( 0.000000000000000000, 1.000000000000000000, 0.000000000000000000 ) ) ;
#10841=ORIENTED_EDGE ( 'NONE', *, *, #11667, .F. ) ;
#10853=EDGE_CURVE ( 'NONE', #1480, #8937, #15236, .T. ) ;
#10869=LINE ( 'NONE', #7766, #2796 ) ;
#10875=ORIENTED_EDGE ( 'NONE', *, *, #5220, .T. ) ;
#10911=CIRCLE ( 'NONE', #1371, 0.7950200000000000600 ) ;
#10917=VERTEX_POINT ( 'NONE', #17648 ) ;
#10927=VERTEX_POINT ( 'NONE', #9232 ) ;
#10928=DIRECTION ( 'NONE',  ( 0.8609107660235850723, 0.000000000000000000, -0.5087559856598092844 ) ) ;
#10933=ORIENTED_EDGE ( 'NONE', *, *, #5621, .T. ) ;
#10947=DIRECTION ( 'NONE',  ( 0.000000000000000000, -1.000000000000000000, 0.000000000000000000 ) ) ;
#10949=CIRCLE ( 'NONE', #17291, 2.182812499999999378 ) ;
#10963=CARTESIAN_POINT ( 'NONE',  ( 2.492193568723835462, 25.39269750000000059, -24.56873394466936134 ) ) ;
#10975=AXIS2_PLACEMENT_3D ( 'NONE', #18021, #15951, #2552 ) ;
#10977=CARTESIAN_POINT ( 'NONE',  ( 1.998220421679061776, 25.39269750000000059, -22.64748046904500356 ) ) ;
#10979=ORIENTED_EDGE ( 'NONE', *, *, #7537, .F. ) ;
#11020=DIRECTION ( 'NONE',  ( 0.000000000000000000, 1.000000000000000000, 0.000000000000000000 ) ) ;
#11028=EDGE_CURVE ( 'NONE', #18192, #12175, #16539, .T. ) ;
#11042=STYLED_ITEM ( 'NONE', ( #2756 ), #21013 ) ;
#11052=FILL_AREA_STYLE_COLOUR ( '', #13894 ) ;
#11054=ORIENTED_EDGE ( 'NONE', *, *, #18177, .T. ) ;
#11082=FACE_OUTER_BOUND ( 'NONE', #12227, .T. ) ;
#11086=EDGE_CURVE ( 'NONE', #21183, #20725, #16326, .T. ) ;
#11090=LINE ( 'NONE', #9526, #20163 ) ;
#11095=ORIENTED_EDGE ( 'NONE', *, *, #13204, .T. ) ;
#11100=FACE_OUTER_BOUND ( 'NONE', #18712, .T. ) ;
#11109=VECTOR ( 'NONE', #15301, 1000.000000000000114 ) ;
#11131=EDGE_CURVE ( 'NONE', #5927, #14184, #3375, .T. ) ;
#11135=CARTESIAN_POINT ( 'NONE',  ( 8.505511374756364873, 24.59767750000000319, -20.97439202360551747 ) ) ;
#11150=CARTESIAN_POINT ( 'NONE',  ( 7.241402720468077092, 25.39269750000000059, -19.25049230170216319 ) ) ;
#11158=CARTESIAN_POINT ( 'NONE',  ( 28.87608719841374949, 40.07707250000000698, -15.73691681567849976 ) ) ;
#11161=ORIENTED_EDGE ( 'NONE', *, *, #9890, .T. ) ;
#11164=DIRECTION ( 'NONE',  ( 0.9685006480810791629, 0.000000000000000000, 0.2490110332224850231 ) ) ;
#11174=CARTESIAN_POINT ( 'NONE',  ( 24.26606285357373594, 28.96330250000000461, -16.92219937337620195 ) ) ;
#11210=DIRECTION ( 'NONE',  ( -0.8609107660235850723, 0.000000000000000000, 0.5087559856598092844 ) ) ;
#11221=DIRECTION ( 'NONE',  ( -0.2490110332224850231, 0.000000000000000000, 0.9685006480810791629 ) ) ;
#11235=CARTESIAN_POINT ( 'NONE',  ( 28.38195592936287781, 1.975802500000001904, -13.81504834214261024 ) ) ;
#11282=CARTESIAN_POINT ( 'NONE',  ( -3.037751992662818257, 28.56769750000000130, -30.02724401157551526 ) ) ;
#11318=CARTESIAN_POINT ( 'NONE',  ( 24.36723594150488026, 39.28205249999999893, 1.799757394719970982 ) ) ;
#11337=ORIENTED_EDGE ( 'NONE', *, *, #17995, .F. ) ;
#11346=CARTESIAN_POINT ( 'NONE',  ( -5.863861779363051419, 34.12394749999999988, -34.80955303575778714 ) ) ;
#11347=DIRECTION ( 'NONE',  ( 0.000000000000000000, 1.000000000000000000, 0.000000000000000000 ) ) ;
#11351=VECTOR ( 'NONE', #12873, 1000.000000000000114 ) ;
#11373=DIRECTION ( 'NONE',  ( 0.2490110332224850509, 0.000000000000000000, -0.9685006480810792739 ) ) ;
#11379=CARTESIAN_POINT ( 'NONE',  ( -39.34028892251012621, 33.32892749999999893, -14.58007324542170480 ) ) ;
#11396=VECTOR ( 'NONE', #20968, 1000.000000000000114 ) ;
#11414=DIRECTION ( 'NONE',  ( 0.000000000000000000, 1.000000000000000000, 0.000000000000000000 ) ) ;
#11435=CARTESIAN_POINT ( 'NONE',  ( 29.64606458365116737, 30.55334249999999940, -15.53894806404596096 ) ) ;
#11448=ORIENTED_EDGE ( 'NONE', *, *, #10097, .F. ) ;
#11452=LINE ( 'NONE', #11881, #6859 ) ;
#11457=ADVANCED_FACE ( 'NONE', ( #7837 ), #21321, .T. ) ;
#11500=LINE ( 'NONE', #13185, #7939 ) ;
#11503=VERTEX_POINT ( 'NONE', #18442 ) ;
#11505=CARTESIAN_POINT ( 'NONE',  ( 1.532169971477637782, 34.03012968715594866, -20.71839214105750315 ) ) ;
#11529=FACE_OUTER_BOUND ( 'NONE', #4383, .T. ) ;
#11553=CARTESIAN_POINT ( 'NONE',  ( 2.417820406479087580, -0.9589899600121986056, -22.53959718991430350 ) ) ;
#11561=AXIS2_PLACEMENT_3D ( 'NONE', #17111, #12355, #15574 ) ;
#11596=VERTEX_POINT ( 'NONE', #18331 ) ;
#11617=CARTESIAN_POINT ( 'NONE',  ( 15.23205103213198441, 19.43957250000000059, -19.24493258192747902 ) ) ;
#11627=DIRECTION ( 'NONE',  ( 0.9685006480810792739, -0.000000000000000000, 0.2490110332224850509 ) ) ;
#11642=CIRCLE ( 'NONE', #12706, 0.7950200000000006151 ) ;
#11652=EDGE_CURVE ( 'NONE', #5927, #19979, #8802, .T. ) ;
#11658=VERTEX_POINT ( 'NONE', #415 ) ;
#11659=AXIS2_PLACEMENT_3D ( 'NONE', #7862, #6420, #14639 ) ;
#11667=EDGE_CURVE ( 'NONE', #10917, #21188, #15258, .T. ) ;
#11681=B_SPLINE_CURVE_WITH_KNOTS ( 'NONE', 3,
 ( #17216, #17114, #192, #2291 ),
 .UNSPECIFIED., .F., .F.,
 ( 4, 4 ),
 ( 0.000000000000000000, 1.000000000000000000 ),
 .UNSPECIFIED. ) ;
#11682=ORIENTED_EDGE ( 'NONE', *, *, #10577, .F. ) ;
#11684=AXIS2_PLACEMENT_3D ( 'NONE', #5949, #19002, #17578 ) ;
#11698=EDGE_CURVE ( 'NONE', #1762, #20415, #6721, .T. ) ;
#11705=DIRECTION ( 'NONE',  ( -0.9685006480810791629, 0.000000000000000000, -0.2490110332224850509 ) ) ;
#11707=ORIENTED_EDGE ( 'NONE', *, *, #8549, .F. ) ;
#11709=VECTOR ( 'NONE', #15500, 1000.000000000000114 ) ;
#11723=CIRCLE ( 'NONE', #6435, 1.587499999999998579 ) ;
#11725=DIRECTION ( 'NONE',  ( -0.8609107660235849613, 0.000000000000000000, 0.5087559856598092844 ) ) ;
#11749=CARTESIAN_POINT ( 'NONE',  ( 0.7843704457339527591, 34.12394749999999988, -23.55949434567611078 ) ) ;
#11757=LINE ( 'NONE', #14871, #1496 ) ;
#11770=DIRECTION ( 'NONE',  ( -0.9685006480810791629, 0.000000000000000000, -0.2490110332224850509 ) ) ;
#11803=VERTEX_POINT ( 'NONE', #3849 ) ;
#11824=CARTESIAN_POINT ( 'NONE',  ( 2.520748753591570690, 25.39269750000000059, -24.56335908395234924 ) ) ;
#11827=VERTEX_POINT ( 'NONE', #1740 ) ;
#11842=LINE ( 'NONE', #15286, #16671 ) ;
#11848=ORIENTED_EDGE ( 'NONE', *, *, #19377, .T. ) ;
#11881=CARTESIAN_POINT ( 'NONE',  ( 16.85197508397059707, 19.43957250000000059, -16.77951971243562923 ) ) ;
#11884=EDGE_CURVE ( 'NONE', #10927, #10018, #19534, .T. ) ;
#11895=ORIENTED_EDGE ( 'NONE', *, *, #17551, .F. ) ;
#11911=FACE_OUTER_BOUND ( 'NONE', #20306, .T. ) ;
#11927=EDGE_CURVE ( 'NONE', #1721, #20753, #10911, .T. ) ;
#11937=ORIENTED_EDGE ( 'NONE', *, *, #19993, .T. ) ;
#11942=DIRECTION ( 'NONE',  ( -0.9488823340533351081, 0.2002559181062071036, -0.2439669719140995230 ) ) ;
#11968=LINE ( 'NONE', #18699, #10242 ) ;
#12005=AXIS2_PLACEMENT_3D ( 'NONE', #903, #17830, #16279 ) ;
#12011=ORIENTED_EDGE ( 'NONE', *, *, #8149, .F. ) ;
#12022=DIRECTION ( 'NONE',  ( 0.000000000000000000, -1.000000000000000000, 0.000000000000000000 ) ) ;
#12038=CARTESIAN_POINT ( 'NONE',  ( 23.77193158452286781, 29.75832250000000201, -15.00033089984030887 ) ) ;
#12044=VECTOR ( 'NONE', #1601, 1000.000000000000114 ) ;
#12066=CARTESIAN_POINT ( 'NONE',  ( 1.998220421679061776, 25.39269750000000059, -22.64748046904500356 ) ) ;
#12067=AXIS2_PLACEMENT_3D ( 'NONE', #1874, #15609, #8620 ) ;
#12078=VECTOR ( 'NONE', #1196, 1000.000000000000114 ) ;
#12081=DIRECTION ( 'NONE',  ( 0.8609107660235850723, 0.000000000000000000, -0.5087559856598092844 ) ) ;
#12095=CARTESIAN_POINT ( 'NONE',  ( 29.15193331460030279, -7.547927499999999235, -13.61707959051006966 ) ) ;
#12117=CARTESIAN_POINT ( 'NONE',  ( -4.728951812473551897, 28.56769750000000130, -29.02782796843600011 ) ) ;
#12134=CIRCLE ( 'NONE', #2951, 0.7950200000000003930 ) ;
#12139=CARTESIAN_POINT ( 'NONE',  ( -5.863861779363051419, 34.12394749999999988, -34.80955303575778714 ) ) ;
#12143=ORIENTED_EDGE ( 'NONE', *, *, #2239, .F. ) ;
#12145=CARTESIAN_POINT ( 'NONE',  ( 8.011380105705496746, 39.28205249999999893, -19.05252355006962617 ) ) ;
#12151=ORIENTED_EDGE ( 'NONE', *, *, #83, .T. ) ;
#12165=FACE_OUTER_BOUND ( 'NONE', #18781, .T. ) ;
#12166=FACE_OUTER_BOUND ( 'NONE', #21765, .T. ) ;
#12168=LINE ( 'NONE', #17244, #13705 ) ;
#12169=EDGE_LOOP ( 'NONE', ( #7364, #1541, #11054, #17876 ) ) ;
#12175=VERTEX_POINT ( 'NONE', #8000 ) ;
#12201=DIRECTION ( 'NONE',  ( 0.000000000000000000, -1.000000000000000000, 0.000000000000000000 ) ) ;
#12204=LINE ( 'NONE', #20580, #3941 ) ;
#12210=CARTESIAN_POINT ( 'NONE',  ( 1.416441012474776606, -1.564831550500477730, -20.74814719358344917 ) ) ;
#12227=EDGE_LOOP ( 'NONE', ( #631, #6933, #9692, #13030 ) ) ;
#12236=FACE_OUTER_BOUND ( 'NONE', #750, .T. ) ;
#12238=CARTESIAN_POINT ( 'NONE',  ( 8.505511374756364873, 34.12394749999999988, -20.97439202360551747 ) ) ;
#12274=ORIENTED_EDGE ( 'NONE', *, *, #7459, .T. ) ;
#12308=DIRECTION ( 'NONE',  ( 0.2490110332224850509, 0.000000000000000000, -0.9685006480810792739 ) ) ;
#12337=DIRECTION ( 'NONE',  ( -0.2490110332224850509, 0.000000000000000000, 0.9685006480810792739 ) ) ;
#12355=DIRECTION ( 'NONE',  ( 0.2490110332224850509, 0.000000000000000000, -0.9685006480810792739 ) ) ;
#12360=DIRECTION ( 'NONE',  ( -0.000000000000000000, 1.000000000000000000, 0.000000000000000000 ) ) ;
#12361=AXIS2_PLACEMENT_3D ( 'NONE', #20123, #794, #7541 ) ;
#12375=ORIENTED_EDGE ( 'NONE', *, *, #492, .T. ) ;
#12380=ADVANCED_FACE ( 'NONE', ( #15424 ), #1585, .T. ) ;
#12385=DIRECTION ( 'NONE',  ( -0.2490110332224850509, 0.000000000000000000, 0.9685006480810792739 ) ) ;
#12392=CARTESIAN_POINT ( 'NONE',  ( -0.8970842057359728061, 34.12394749999999988, -22.54358764576276286 ) ) ;
#12394=ORIENTED_EDGE ( 'NONE', *, *, #14198, .T. ) ;
#12414=PLANE ( 'NONE',  #18845 ) ;
#12445=VECTOR ( 'NONE', #18871, 1000.000000000000000 ) ;
#12457=DIRECTION ( 'NONE',  ( 0.000000000000000000, 1.000000000000000000, 0.000000000000000000 ) ) ;
#12469=VERTEX_POINT ( 'NONE', #21325 ) ;
#12488=ORIENTED_EDGE ( 'NONE', *, *, #8549, .T. ) ;
#12492=ORIENTED_EDGE ( 'NONE', *, *, #3670, .F. ) ;
#12502=CARTESIAN_POINT ( 'NONE',  ( -6.100806958595617502, 34.12394749999684507, -35.21050882107662972 ) ) ;
#12505=DIRECTION ( 'NONE',  ( 0.9685006480810787188, 0.000000000000000000, 0.2490110332224867162 ) ) ;
#12507=DIRECTION ( 'NONE',  ( -0.5087559856598098396, 0.000000000000000000, -0.8609107660235847392 ) ) ;
#12517=VERTEX_POINT ( 'NONE', #6071 ) ;
#12531=DIRECTION ( 'NONE',  ( -0.8609107660235848503, 0.000000000000000000, 0.5087559856598096175 ) ) ;
#12550=DIRECTION ( 'NONE',  ( 0.2490110332224850509, 0.000000000000000000, -0.9685006480810792739 ) ) ;
#12551=CARTESIAN_POINT ( 'NONE',  ( -5.863861779363051419, -1.594802499999999013, -34.80955303575778714 ) ) ;
#12571=ORIENTED_EDGE ( 'NONE', *, *, #15186, .T. ) ;
#12602=ORIENTED_EDGE ( 'NONE', *, *, #7315, .T. ) ;
#12605=CARTESIAN_POINT ( 'NONE',  ( 0.2641497867371597752, 25.39269750000000059, -24.43980549416641068 ) ) ;
#12621=DIRECTION ( 'NONE',  ( 0.000000000000000000, 1.000000000000000000, 0.000000000000000000 ) ) ;
#12647=CARTESIAN_POINT ( 'NONE',  ( 28.38195592936287781, 29.75832250000000201, -13.81504834214261024 ) ) ;
#12662=CARTESIAN_POINT ( 'NONE',  ( 29.64606458365116737, -6.752907499999998286, -15.53894806404596096 ) ) ;
#12663=ORIENTED_EDGE ( 'NONE', *, *, #18070, .F. ) ;
#12675=LINE ( 'NONE', #20960, #9904 ) ;
#12679=DIRECTION ( 'NONE',  ( 0.000000000000000000, 1.000000000000000000, 0.000000000000000000 ) ) ;
#12681=VERTEX_POINT ( 'NONE', #10151 ) ;
#12686=LINE ( 'NONE', #4281, #3799 ) ;
#12699=ORIENTED_EDGE ( 'NONE', *, *, #11698, .T. ) ;
#12706=AXIS2_PLACEMENT_3D ( 'NONE', #10268, #3206, #18459 ) ;
#12716=ORIENTED_EDGE ( 'NONE', *, *, #10097, .T. ) ;
#12726=PLANE ( 'NONE',  #3207 ) ;
#12730=VECTOR ( 'NONE', #17298, 1000.000000000000114 ) ;
#12752=ORIENTED_EDGE ( 'NONE', *, *, #19487, .T. ) ;
#12771=EDGE_CURVE ( 'NONE', #18859, #20415, #1649, .T. ) ;
#12782=CARTESIAN_POINT ( 'NONE',  ( 8.011380105705496746, -6.752907499999998286, -19.05252355006962617 ) ) ;
#12794=LINE ( 'NONE', #19517, #10647 ) ;
#12795=CLOSED_SHELL ( 'NONE', ( #18839, #762, #9475, #10731, #15921, #2842, #20729, #19231, #12380, #15515, #20571, #15464, #4244, #21524, #21552, #1537, #6882, #7105, #17759, #18220, #21371, #16167, #21379, #5995, #16134, #15513, #9194, #15136, #21579, #20869, #11457, #3860, #1290, #12943, #16000, #15871, #167, #10468, #15627, #5197, #14946, #8896, #19880, #3747, #10548, #5974, #17755, #17462, #17700, #1336, #8463, #8693, #3866, #7056, #5656, #4980 ) ) ;
#12797=AXIS2_PLACEMENT_3D ( 'NONE', #6072, #7526, #4433 ) ;
#12802=ORIENTED_EDGE ( 'NONE', *, *, #2791, .T. ) ;
#12812=ORIENTED_EDGE ( 'NONE', *, *, #16138, .F. ) ;
#12813=VECTOR ( 'NONE', #18594, 1000.000000000000114 ) ;
#12816=CARTESIAN_POINT ( 'NONE',  ( 28.87608719841374949, 29.75832250000000201, -15.73691681567849976 ) ) ;
#12824=VECTOR ( 'NONE', #15910, 1000.000000000000114 ) ;
#12828=AXIS2_PLACEMENT_3D ( 'NONE', #14661, #21367, #4686 ) ;
#12844=CARTESIAN_POINT ( 'NONE',  ( 1.670997140563193373, -1.594802499999999013, -22.76294857149378714 ) ) ;
#12847=ORIENTED_EDGE ( 'NONE', *, *, #4771, .T. ) ;
#12849=DIRECTION ( 'NONE',  ( -0.8558687090795834562, 0.000000000000000000, 0.5171931484643310650 ) ) ;
#12852=CIRCLE ( 'NONE', #2944, 1.587499999999998579 ) ;
#12865=CARTESIAN_POINT ( 'NONE',  ( 29.64606458365116737, -6.752907499999998286, -15.53894806404596096 ) ) ;
#12872=AXIS2_PLACEMENT_3D ( 'NONE', #20994, #18888, #13952 ) ;
#12873=DIRECTION ( 'NONE',  ( -0.9685006480810791629, 4.068963411654120556E-16, -0.2490110332224850231 ) ) ;
#12874=EDGE_CURVE ( 'NONE', #4408, #21155, #19343, .T. ) ;
#12894=VECTOR ( 'NONE', #10081, 1000.000000000000114 ) ;
#12897=EDGE_CURVE ( 'NONE', #21869, #4861, #20713, .T. ) ;
#12905=ORIENTED_EDGE ( 'NONE', *, *, #15321, .T. ) ;
#12913=ORIENTED_EDGE ( 'NONE', *, *, #15186, .F. ) ;
#12923=ORIENTED_EDGE ( 'NONE', *, *, #15321, .F. ) ;
#12943=ADVANCED_FACE ( 'NONE', ( #11911 ), #15366, .F. ) ;
#12949=SURFACE_STYLE_USAGE ( .BOTH. , #4313 ) ;
#12955=CYLINDRICAL_SURFACE ( 'NONE', #12797, 0.7950200000000005041 ) ;
#12964=DIRECTION ( 'NONE',  ( 0.2490110332224850231, 0.000000000000000000, -0.9685006480810791629 ) ) ;
#12987=CIRCLE ( 'NONE', #13347, 1.587500000000000355 ) ;
#12994=PLANE ( 'NONE',  #462 ) ;
#13005=EDGE_CURVE ( 'NONE', #11503, #7489, #19661, .T. ) ;
#13016=CARTESIAN_POINT ( 'NONE',  ( 22.05855709630448303, 26.98019749999999917, -44.85793026951184004 ) ) ;
#13022=EDGE_CURVE ( 'NONE', #1096, #20415, #17327, .T. ) ;
#13030=ORIENTED_EDGE ( 'NONE', *, *, #18597, .F. ) ;
#13033=FACE_OUTER_BOUND ( 'NONE', #5288, .T. ) ;
#13059=ORIENTED_EDGE ( 'NONE', *, *, #11028, .F. ) ;
#13061=DIRECTION ( 'NONE',  ( 0.000000000000000000, -1.000000000000000000, 0.000000000000000000 ) ) ;
#13066=EDGE_CURVE ( 'NONE', #2577, #4289, #12987, .T. ) ;
#13078=ORIENTED_EDGE ( 'NONE', *, *, #11652, .F. ) ;
#13102=CARTESIAN_POINT ( 'NONE',  ( 0.7843704457339527591, -1.594802499999999013, -23.55949434567611078 ) ) ;
#13135=ORIENTED_EDGE ( 'NONE', *, *, #478, .F. ) ;
#13142=DIRECTION ( 'NONE',  ( -0.9685006480810791629, 0.000000000000000000, -0.2490110332224850231 ) ) ;
#13177=EDGE_CURVE ( 'NONE', #15380, #12517, #12686, .T. ) ;
#13185=CARTESIAN_POINT ( 'NONE',  ( 28.38195592936287781, 40.07707250000000698, -13.81504834214261024 ) ) ;
#13190=CARTESIAN_POINT ( 'NONE',  ( -2.234700160307072192, 26.98019749999999917, -24.80708529208898483 ) ) ;
#13193=EDGE_CURVE ( 'NONE', #5628, #12469, #3158, .T. ) ;
#13198=VECTOR ( 'NONE', #6223, 1000.000000000000114 ) ;
#13204=EDGE_CURVE ( 'NONE', #13546, #16767, #8347, .T. ) ;
#13212=DIRECTION ( 'NONE',  ( 0.000000000000000000, 1.000000000000000000, 0.000000000000000000 ) ) ;
#13219=EDGE_CURVE ( 'NONE', #490, #2577, #18208, .T. ) ;
#13252=VECTOR ( 'NONE', #20651, 1000.000000000000000 ) ;
#13268=CYLINDRICAL_SURFACE ( 'NONE', #7159, 0.7950200000000001710 ) ;
#13279=ORIENTED_EDGE ( 'NONE', *, *, #6461, .F. ) ;
#13282=ORIENTED_EDGE ( 'NONE', *, *, #4272, .F. ) ;
#13293=DIRECTION ( 'NONE',  ( 0.2490110332224850231, 0.000000000000000000, -0.9685006480810791629 ) ) ;
#13303=ORIENTED_EDGE ( 'NONE', *, *, #21261, .F. ) ;
#13307=EDGE_LOOP ( 'NONE', ( #14292, #20865, #5711, #1372 ) ) ;
#13318=EDGE_CURVE ( 'NONE', #6074, #1216, #16968, .T. ) ;
#13326=CARTESIAN_POINT ( 'NONE',  ( 8.505511374756364873, 24.59767750000000319, -20.97439202360551747 ) ) ;
#13347=AXIS2_PLACEMENT_3D ( 'NONE', #21178, #4497, #14582 ) ;
#13354=EDGE_LOOP ( 'NONE', ( #4150, #3075, #2982, #14912 ) ) ;
#13372=AXIS2_PLACEMENT_3D ( 'NONE', #3231, #20116, #4989 ) ;
#13383=DIRECTION ( 'NONE',  ( 0.8609107660235849613, 0.000000000000000000, -0.5087559856598092844 ) ) ;
#13413=PLANE ( 'NONE',  #12361 ) ;
#13428=CARTESIAN_POINT ( 'NONE',  ( -5.536601939709260733, 26.98019749999999917, -30.39452380949970944 ) ) ;
#13454=EDGE_CURVE ( 'NONE', #12175, #2498, #18730, .T. ) ;
#13494=AXIS2_PLACEMENT_3D ( 'NONE', #4188, #10928, #16358 ) ;
#13534=DIRECTION ( 'NONE',  ( 0.9685006480810790519, 0.000000000000000000, 0.2490110332224857170 ) ) ;
#13538=VERTEX_POINT ( 'NONE', #19284 ) ;
#13546=VERTEX_POINT ( 'NONE', #16102 ) ;
#13555=CIRCLE ( 'NONE', #14629, 2.182812500000000711 ) ;
#13561=EDGE_CURVE ( 'NONE', #13546, #5667, #19388, .T. ) ;
#13586=VECTOR ( 'NONE', #3245, 1000.000000000000114 ) ;
#13594=CYLINDRICAL_SURFACE ( 'NONE', #3267, 2.182812499999999378 ) ;
#13605=ORIENTED_EDGE ( 'NONE', *, *, #83, .F. ) ;
#13606=DIRECTION ( 'NONE',  ( 0.4210968886563865587, 0.9005306316452192927, 0.1082681478209225612 ) ) ;
#13609=VECTOR ( 'NONE', #11725, 1000.000000000000114 ) ;
#13618=ORIENTED_EDGE ( 'NONE', *, *, #13454, .F. ) ;
#13627=EDGE_LOOP ( 'NONE', ( #15832, #6792, #10613, #14672, #663, #16607 ) ) ;
#13628=ORIENTED_EDGE ( 'NONE', *, *, #17995, .T. ) ;
#13645=DIRECTION ( 'NONE',  ( 0.2490110332224850509, 0.000000000000000000, -0.9685006480810792739 ) ) ;
#13662=VERTEX_POINT ( 'NONE', #12662 ) ;
#13673=ORIENTED_EDGE ( 'NONE', *, *, #19487, .F. ) ;
#13677=DIRECTION ( 'NONE',  ( -0.2490110332224850509, 0.000000000000000000, 0.9685006480810792739 ) ) ;
#13687=LINE ( 'NONE', #18745, #2605 ) ;
#13696=ORIENTED_EDGE ( 'NONE', *, *, #20646, .F. ) ;
#13700=CARTESIAN_POINT ( 'NONE',  ( -3.042350287543033716, 2.373947500000000765, -26.17378113315171007 ) ) ;
#13705=VECTOR ( 'NONE', #13955, 1000.000000000000000 ) ;
#13710=EDGE_LOOP ( 'NONE', ( #16472, #17475, #4620, #8732, #14372, #9104 ) ) ;
#13736=EDGE_CURVE ( 'NONE', #18192, #6074, #9203, .T. ) ;
#13752=CARTESIAN_POINT ( 'NONE',  ( 8.011380105705496746, -1.594802499999999013, -19.05252355006962617 ) ) ;
#13771=ORIENTED_EDGE ( 'NONE', *, *, #17786, .T. ) ;
#13773=AXIS2_PLACEMENT_3D ( 'NONE', #11174, #14630, #9403 ) ;
#13783=EDGE_LOOP ( 'NONE', ( #18013, #20641, #12602, #17669, #20108, #19074, #17677, #7663 ) ) ;
#13813=ORIENTED_EDGE ( 'NONE', *, *, #12771, .F. ) ;
#13822=ORIENTED_EDGE ( 'NONE', *, *, #20904, .T. ) ;
#13832=CARTESIAN_POINT ( 'NONE',  ( 8.505511374756364873, 6.343967500000000648, -20.97439202360551747 ) ) ;
#13842=VERTEX_POINT ( 'NONE', #8324 ) ;
#13863=APPLICATION_CONTEXT ( 'automotive_design' ) ;
#13872=FACE_OUTER_BOUND ( 'NONE', #5493, .T. ) ;
#13880=CARTESIAN_POINT ( 'NONE',  ( 7.735533989518945219, 24.59767750000000319, -21.17236077523805449 ) ) ;
#13894=COLOUR_RGB ( '', 0.31764706, 0.68627451, 0.89019608) ;
#13920=VECTOR ( 'NONE', #5489, 1000.000000000000114 ) ;
#13924=EDGE_CURVE ( 'NONE', #3406, #6199, #17167, .T. ) ;
#13941=ORIENTED_EDGE ( 'NONE', *, *, #14688, .T. ) ;
#13945=VERTEX_POINT ( 'NONE', #18491 ) ;
#13952=DIRECTION ( 'NONE',  ( -0.8609107660235848503, 0.000000000000000000, 0.5087559856598096175 ) ) ;
#13955=DIRECTION ( 'NONE',  ( 0.000000000000000000, 1.000000000000000000, 0.000000000000000000 ) ) ;
#13960=LINE ( 'NONE', #5190, #7123 ) ;
#13987=CARTESIAN_POINT ( 'NONE',  ( 28.87608719841374949, -6.752907499999998286, -15.73691681567849976 ) ) ;
#13993=DIRECTION ( 'NONE',  ( 0.2490110332224850509, 0.000000000000000000, -0.9685006480810792739 ) ) ;
#14018=CARTESIAN_POINT ( 'NONE',  ( 4.936390548048069427, 34.12394749999999988, -19.84313358055101517 ) ) ;
#14022=CARTESIAN_POINT ( 'NONE',  ( 0.000000000000000000, 0.000000000000000000, 0.000000000000000000 ) ) ;
#14036=CARTESIAN_POINT ( 'NONE',  ( -5.132424380828760846, 25.39269750000000059, -7.958392962111297209 ) ) ;
#14040=ORIENTED_EDGE ( 'NONE', *, *, #16267, .T. ) ;
#14041=VERTEX_POINT ( 'NONE', #5664 ) ;
#14050=AXIS2_PLACEMENT_3D ( 'NONE', #2289, #20626, #20738 ) ;
#14059=CIRCLE ( 'NONE', #7693, 3.970020000000000326 ) ;
#14063=PLANE ( 'NONE',  #11684 ) ;
#14066=ORIENTED_EDGE ( 'NONE', *, *, #19798, .F. ) ;
#14076=LINE ( 'NONE', #8963, #8400 ) ;
#14125=CARTESIAN_POINT ( 'NONE',  ( 8.505511374756364873, 39.28205249999999893, -20.97439202360551747 ) ) ;
#14130=EDGE_LOOP ( 'NONE', ( #19932, #4093, #9062, #19405 ) ) ;
#14152=ORIENTED_EDGE ( 'NONE', *, *, #157, .T. ) ;
#14176=DIRECTION ( 'NONE',  ( -0.8609107660235850723, 0.000000000000000000, 0.5087559856598092844 ) ) ;
#14178=EDGE_LOOP ( 'NONE', ( #4455, #14722, #17582, #18338 ) ) ;
#14184=VERTEX_POINT ( 'NONE', #21454 ) ;
#14198=EDGE_CURVE ( 'NONE', #14184, #18623, #18547, .T. ) ;
#14232=VERTEX_POINT ( 'NONE', #21348 ) ;
#14236=VERTEX_POINT ( 'NONE', #18159 ) ;
#14242=ORIENTED_EDGE ( 'NONE', *, *, #20870, .F. ) ;
#14272=ORIENTED_EDGE ( 'NONE', *, *, #21680, .T. ) ;
#14289=DIRECTION ( 'NONE',  ( 0.9685006480810790519, 0.000000000000000000, 0.2490110332224857170 ) ) ;
#14292=ORIENTED_EDGE ( 'NONE', *, *, #19882, .F. ) ;
#14305=FACE_OUTER_BOUND ( 'NONE', #3486, .T. ) ;
#14308=CARTESIAN_POINT ( 'NONE',  ( 29.64606458365116737, -7.547927499999999235, -15.53894806404596096 ) ) ;
#14313=ORIENTED_EDGE ( 'NONE', *, *, #19826, .T. ) ;
#14337=AXIS2_PLACEMENT_3D ( 'NONE', #13987, #13645, #13534 ) ;
#14339=ORIENTED_EDGE ( 'NONE', *, *, #2788, .T. ) ;
#14345=ORIENTED_EDGE ( 'NONE', *, *, #3670, .T. ) ;
#14359=CARTESIAN_POINT ( 'NONE',  ( 23.77193158452286781, 3.565842500000000914, -15.00033089984030887 ) ) ;
#14372=ORIENTED_EDGE ( 'NONE', *, *, #10577, .T. ) ;
#14376=FACE_OUTER_BOUND ( 'NONE', #10226, .T. ) ;
#14377=FACE_OUTER_BOUND ( 'NONE', #911, .T. ) ;
#14381=LINE ( 'NONE', #14489, #15978 ) ;
#14411=CYLINDRICAL_SURFACE ( 'NONE', #20511, 0.7950200000000005041 ) ;
#14433=CARTESIAN_POINT ( 'NONE',  ( 16.85197508397059707, 19.43957250000000059, -16.77951971243562923 ) ) ;
#14439=( GEOMETRIC_REPRESENTATION_CONTEXT ( 3 ) GLOBAL_UNCERTAINTY_ASSIGNED_CONTEXT ( ( #18729 ) ) GLOBAL_UNIT_ASSIGNED_CONTEXT ( ( #8229, #1267, #15105 ) ) REPRESENTATION_CONTEXT ( 'NONE', 'WORKASPACE' ) );
#14453=FACE_OUTER_BOUND ( 'NONE', #19120, .T. ) ;
#14462=VECTOR ( 'NONE', #195, 1000.000000000000000 ) ;
#14463=VERTEX_POINT ( 'NONE', #20582 ) ;
#14489=CARTESIAN_POINT ( 'NONE',  ( 29.15193331460030279, 39.28205249999999893, -13.61707959051006966 ) ) ;
#14497=FACE_OUTER_BOUND ( 'NONE', #13307, .T. ) ;
#14499=ORIENTED_EDGE ( 'NONE', *, *, #19795, .F. ) ;
#14508=EDGE_CURVE ( 'NONE', #10511, #513, #8541, .T. ) ;
#14528=ORIENTED_EDGE ( 'NONE', *, *, #16291, .F. ) ;
#14546=DIRECTION ( 'NONE',  ( -0.9685006480810791629, 0.000000000000000000, -0.2490110332224850231 ) ) ;
#14575=AXIS2_PLACEMENT_3D ( 'NONE', #8076, #20106, #11942 ) ;
#14579=APPLICATION_CONTEXT ( 'automotive_design' ) ;
#14582=DIRECTION ( 'NONE',  ( 0.000000000000000000, 1.000000000000000000, 0.000000000000000000 ) ) ;
#14584=ORIENTED_EDGE ( 'NONE', *, *, #2598, .F. ) ;
#14588=VECTOR ( 'NONE', #1154, 1000.000000000000227 ) ;
#14595=ORIENTED_EDGE ( 'NONE', *, *, #20065, .F. ) ;
#14609=CARTESIAN_POINT ( 'NONE',  ( 8.505511374756364873, 36.49567249999999774, -20.97439202360551747 ) ) ;
#14629=AXIS2_PLACEMENT_3D ( 'NONE', #1180, #2627, #6257 ) ;
#14630=DIRECTION ( 'NONE',  ( -0.2490110332224850509, 0.000000000000000000, 0.9685006480810792739 ) ) ;
#14639=DIRECTION ( 'NONE',  ( 0.5087559856598089514, 0.000000000000000000, 0.8609107660235851833 ) ) ;
#14661=CARTESIAN_POINT ( 'NONE',  ( -7.949728765565600597, -7.547927499999999235, -34.47798802950714503 ) ) ;
#14672=ORIENTED_EDGE ( 'NONE', *, *, #4538, .F. ) ;
#14680=AXIS2_PLACEMENT_3D ( 'NONE', #875, #547, #8826 ) ;
#14688=EDGE_CURVE ( 'NONE', #14463, #17254, #10869, .T. ) ;
#14707=ORIENTED_EDGE ( 'NONE', *, *, #18705, .F. ) ;
#14716=ORIENTED_EDGE ( 'NONE', *, *, #14508, .F. ) ;
#14719=LINE ( 'NONE', #11158, #8200 ) ;
#14722=ORIENTED_EDGE ( 'NONE', *, *, #21851, .F. ) ;
#14729=VERTEX_POINT ( 'NONE', #10977 ) ;
#14733=CARTESIAN_POINT ( 'NONE',  ( 1.923689137428217455, 33.48813496001219647, -20.61772871637841220 ) ) ;
#14735=CARTESIAN_POINT ( 'NONE',  ( 29.15193331460030279, -7.547927499999999235, -13.61707959051006966 ) ) ;
#14772=ORIENTED_EDGE ( 'NONE', *, *, #7995, .F. ) ;
#14773=DIRECTION ( 'NONE',  ( 0.9685006480810791629, 0.000000000000000000, 0.2490110332224850231 ) ) ;
#14784=DIRECTION ( 'NONE',  ( -0.8609107660235849613, 0.000000000000000000, 0.5087559856598092844 ) ) ;
#14790=EDGE_CURVE ( 'NONE', #1480, #7489, #4126, .T. ) ;
#14800=DIRECTION ( 'NONE',  ( -0.2490110332224850509, 0.000000000000000000, 0.9685006480810792739 ) ) ;
#14824=VECTOR ( 'NONE', #17615, 1000.000000000000114 ) ;
#14827=ORIENTED_EDGE ( 'NONE', *, *, #2050, .T. ) ;
#14831=ORIENTED_EDGE ( 'NONE', *, *, #5817, .F. ) ;
#14842=FACE_OUTER_BOUND ( 'NONE', #425, .T. ) ;
#14864=EDGE_CURVE ( 'NONE', #8797, #4861, #3230, .T. ) ;
#14868=CARTESIAN_POINT ( 'NONE',  ( -0.5435003404963313356, 3.961447500000001565, -25.80650133522849998 ) ) ;
#14871=CARTESIAN_POINT ( 'NONE',  ( 28.87608719841374949, 2.770822500000000854, -15.73691681567849976 ) ) ;
#14872=LINE ( 'NONE', #19603, #13586 ) ;
#14912=ORIENTED_EDGE ( 'NONE', *, *, #21707, .T. ) ;
#14939=LINE ( 'NONE', #3088, #17334 ) ;
#14946=ADVANCED_FACE ( 'NONE', ( #6212 ), #14975, .F. ) ;
#14950=VECTOR ( 'NONE', #7020, 1000.000000000000114 ) ;
#14951=AXIS2_PLACEMENT_3D ( 'NONE', #17295, #16098, #19278 ) ;
#14957=LINE ( 'NONE', #21671, #13609 ) ;
#14963=DIRECTION ( 'NONE',  ( 0.2490110332224850509, 0.000000000000000000, -0.9685006480810792739 ) ) ;
#14970=VERTEX_POINT ( 'NONE', #9639 ) ;
#14975=PLANE ( 'NONE',  #20084 ) ;
#15016=CARTESIAN_POINT ( 'NONE',  ( 13.11799571124250363, 13.08957250000000094, -19.78847697788343396 ) ) ;
#15054=ORIENTED_EDGE ( 'NONE', *, *, #16578, .T. ) ;
#15061=CARTESIAN_POINT ( 'NONE',  ( -7.949728765565600597, 33.32892749999999893, -34.47798802950714503 ) ) ;
#15068=CARTESIAN_POINT ( 'NONE',  ( 14.33584040382675262, 6.343967500000000648, -46.84351661546690337 ) ) ;
#15105=( NAMED_UNIT ( * ) SI_UNIT ( $, .STERADIAN. ) SOLID_ANGLE_UNIT ( ) );
#15136=ADVANCED_FACE ( 'NONE', ( #5534 ), #4006, .T. ) ;
#15151=ORIENTED_EDGE ( 'NONE', *, *, #4185, .F. ) ;
#15153=LINE ( 'NONE', #4645, #6377 ) ;
#15168=DIRECTION ( 'NONE',  ( 0.000000000000000000, 1.000000000000000000, 0.000000000000000000 ) ) ;
#15175=ORIENTED_EDGE ( 'NONE', *, *, #6381, .T. ) ;
#15180=EDGE_CURVE ( 'NONE', #5796, #18451, #4541, .T. ) ;
#15186=EDGE_CURVE ( 'NONE', #11827, #13842, #19752, .T. ) ;
#15188=CARTESIAN_POINT ( 'NONE',  ( 28.38195592936287781, -7.547927499999999235, -13.81504834214261024 ) ) ;
#15221=AXIS2_PLACEMENT_3D ( 'NONE', #1717, #1506, #3288 ) ;
#15225=ORIENTED_EDGE ( 'NONE', *, *, #20281, .F. ) ;
#15226=ORIENTED_EDGE ( 'NONE', *, *, #13736, .T. ) ;
#15235=EDGE_CURVE ( 'NONE', #2495, #4521, #11642, .T. ) ;
#15236=LINE ( 'NONE', #5150, #6639 ) ;
#15238=CIRCLE ( 'NONE', #5000, 0.7950200000000003930 ) ;
#15239=ORIENTED_EDGE ( 'NONE', *, *, #19826, .F. ) ;
#15251=VECTOR ( 'NONE', #11164, 1000.000000000000114 ) ;
#15258=LINE ( 'NONE', #13700, #18321 ) ;
#15286=CARTESIAN_POINT ( 'NONE',  ( 8.011380105705496746, -6.752907499999998286, -19.05252355006962617 ) ) ;
#15301=DIRECTION ( 'NONE',  ( -0.2490110332224850231, 0.000000000000000000, 0.9685006480810791629 ) ) ;
#15302=AXIS2_PLACEMENT_3D ( 'NONE', #14308, #17602, #9076 ) ;
#15316=DIRECTION ( 'NONE',  ( 0.9685006480810792739, -0.000000000000000000, 0.2490110332224850509 ) ) ;
#15321=EDGE_CURVE ( 'NONE', #9160, #10315, #5647, .T. ) ;
#15355=VERTEX_POINT ( 'NONE', #21699 ) ;
#15366=CYLINDRICAL_SURFACE ( 'NONE', #14050, 1.983740000000001391 ) ;
#15370=DIRECTION ( 'NONE',  ( 0.9685006480810792739, 0.000000000000000000, 0.2490110332224850509 ) ) ;
#15380=VERTEX_POINT ( 'NONE', #17954 ) ;
#15397=FACE_OUTER_BOUND ( 'NONE', #14130, .T. ) ;
#15410=CARTESIAN_POINT ( 'NONE',  ( 7.735533989518945219, 25.39269750000000059, -21.17236077523805449 ) ) ;
#15417=CARTESIAN_POINT ( 'NONE',  ( 1.202411175319977765, -7.547927499999999235, -22.85209084599881635 ) ) ;
#15424=FACE_OUTER_BOUND ( 'NONE', #808, .T. ) ;
#15446=ORIENTED_EDGE ( 'NONE', *, *, #16908, .F. ) ;
#15464=ADVANCED_FACE ( 'NONE', ( #20567 ), #13413, .T. ) ;
#15475=PLANE ( 'NONE',  #9959 ) ;
#15500=DIRECTION ( 'NONE',  ( -0.5087559856598092844, 0.000000000000000000, -0.8609107660235849613 ) ) ;
#15513=ADVANCED_FACE ( 'NONE', ( #7321 ), #12414, .F. ) ;
#15515=ADVANCED_FACE ( 'NONE', ( #14842 ), #8182, .T. ) ;
#15540=CARTESIAN_POINT ( 'NONE',  ( 1.670997140563193373, 34.12394749999999988, -22.76294857149378714 ) ) ;
#15557=ORIENTED_EDGE ( 'NONE', *, *, #13561, .T. ) ;
#15560=LINE ( 'NONE', #14125, #8904 ) ;
#15562=CYLINDRICAL_SURFACE ( 'NONE', #18726, 1.587500000000002132 ) ;
#15565=ORIENTED_EDGE ( 'NONE', *, *, #19385, .T. ) ;
#15574=DIRECTION ( 'NONE',  ( 0.9685006480810790519, 0.000000000000000000, 0.2490110332224857170 ) ) ;
#15575=EDGE_LOOP ( 'NONE', ( #1938, #17201, #19734, #18183 ) ) ;
#15577=LINE ( 'NONE', #526, #18424 ) ;
#15583=CIRCLE ( 'NONE', #10975, 3.174999999999998490 ) ;
#15585=PLANE ( 'NONE',  #6426 ) ;
#15598=VECTOR ( 'NONE', #942, 1000.000000000000000 ) ;
#15609=DIRECTION ( 'NONE',  ( 0.8609107660235850723, 0.000000000000000000, -0.5087559856598092844 ) ) ;
#15610=CARTESIAN_POINT ( 'NONE',  ( 23.49608546833631451, 3.565842500000000914, -17.12016812500874252 ) ) ;
#15619=CIRCLE ( 'NONE', #2883, 2.182812499999997158 ) ;
#15622=CIRCLE ( 'NONE', #16662, 1.587500000000001688 ) ;
#15626=DIRECTION ( 'NONE',  ( -0.9685006480810792739, 0.000000000000000000, -0.2490110332224850509 ) ) ;
#15627=ADVANCED_FACE ( 'NONE', ( #3328 ), #3426, .F. ) ;
#15644=FACE_BOUND ( 'NONE', #6152, .T. ) ;
#15651=DIRECTION ( 'NONE',  ( -0.2490110332224850509, 0.000000000000000000, 0.9685006480810792739 ) ) ;
#15659=CARTESIAN_POINT ( 'NONE',  ( -6.268352501591477832, -0.7997824999999986195, -35.49402737582407497 ) ) ;
#15689=ORIENTED_EDGE ( 'NONE', *, *, #20065, .T. ) ;
#15698=PLANE ( 'NONE',  #20899 ) ;
#15706=DIRECTION ( 'NONE',  ( -0.000000000000000000, 1.000000000000000000, 0.000000000000000000 ) ) ;
#15711=ORIENTED_EDGE ( 'NONE', *, *, #16039, .F. ) ;
#15712=AXIS2_PLACEMENT_3D ( 'NONE', #215, #10161, #16904 ) ;
#15726=CARTESIAN_POINT ( 'NONE',  ( -1.351150467732365579, 2.373947500000000765, -27.17319717629097653 ) ) ;
#15727=CARTESIAN_POINT ( 'NONE',  ( 29.64606458365116737, -1.985327499999998357, -15.53894806404596096 ) ) ;
#15728=CARTESIAN_POINT ( 'NONE',  ( 28.87608719841374949, -7.547927499999999235, -15.73691681567849976 ) ) ;
#15765=SHAPE_DEFINITION_REPRESENTATION ( #21496, #560 ) ;
#15775=CARTESIAN_POINT ( 'NONE',  ( 22.05855709630448303, 3.961447500000001565, -44.85793026951184004 ) ) ;
#15784=DIRECTION ( 'NONE',  ( -0.000000000000000000, 1.000000000000000000, 0.000000000000000000 ) ) ;
#15815=ORIENTED_EDGE ( 'NONE', *, *, #8029, .T. ) ;
#15820=DIRECTION ( 'NONE',  ( 0.000000000000000000, 1.000000000000000000, 0.000000000000000000 ) ) ;
#15822=CARTESIAN_POINT ( 'NONE',  ( 29.64606458365116737, -7.547927499999999235, -15.53894806404596096 ) ) ;
#15832=ORIENTED_EDGE ( 'NONE', *, *, #6461, .T. ) ;
#15841=DIRECTION ( 'NONE',  ( -0.2490110332224850509, 0.000000000000000000, 0.9685006480810792739 ) ) ;
#15851=DIRECTION ( 'NONE',  ( 0.000000000000000000, 1.000000000000000000, 0.000000000000000000 ) ) ;
#15860=EDGE_CURVE ( 'NONE', #4521, #16037, #21092, .T. ) ;
#15871=ADVANCED_FACE ( 'NONE', ( #14376 ), #4626, .F. ) ;
#15881=VECTOR ( 'NONE', #21791, 1000.000000000000114 ) ;
#15893=PLANE ( 'NONE',  #10620 ) ;
#15910=DIRECTION ( 'NONE',  ( -0.2490110332224850231, 0.000000000000000000, 0.9685006480810791629 ) ) ;
#15914=CARTESIAN_POINT ( 'NONE',  ( 29.15193331460030279, -6.752907499999998286, -13.61707959051006966 ) ) ;
#15921=ADVANCED_FACE ( 'NONE', ( #14453 ), #946, .F. ) ;
#15929=ORIENTED_EDGE ( 'NONE', *, *, #7059, .F. ) ;
#15941=CARTESIAN_POINT ( 'NONE',  ( -3.037751992662818257, 3.961447500000001565, -30.02724401157551526 ) ) ;
#15951=DIRECTION ( 'NONE',  ( -0.2490110332224850509, 0.000000000000000000, 0.9685006480810792739 ) ) ;
#15964=PLANE ( 'NONE',  #15302 ) ;
#15974=CIRCLE ( 'NONE', #18064, 1.587499999999999911 ) ;
#15977=CYLINDRICAL_SURFACE ( 'NONE', #754, 0.7950199999999998379 ) ;
#15978=VECTOR ( 'NONE', #7834, 1000.000000000000114 ) ;
#16000=ADVANCED_FACE ( 'NONE', ( #12236 ), #18961, .F. ) ;
#16014=AXIS2_PLACEMENT_3D ( 'NONE', #15775, #7345, #19049 ) ;
#16015=DIRECTION ( 'NONE',  ( -0.2490110332224850509, 0.000000000000000000, 0.9685006480810792739 ) ) ;
#16031=CYLINDRICAL_SURFACE ( 'NONE', #2864, 0.7950200000000003930 ) ;
#16037=VERTEX_POINT ( 'NONE', #11553 ) ;
#16039=EDGE_CURVE ( 'NONE', #17975, #21188, #16641, .T. ) ;
#16048=CARTESIAN_POINT ( 'NONE',  ( 8.781357490942916399, 39.28205249999999893, -18.85455479843708559 ) ) ;
#16056=VECTOR ( 'NONE', #14784, 1000.000000000000114 ) ;
#16080=AXIS2_PLACEMENT_3D ( 'NONE', #1436, #21443, #16280 ) ;
#16098=DIRECTION ( 'NONE',  ( -0.8609107660235850723, 0.000000000000000000, 0.5087559856598092844 ) ) ;
#16102=CARTESIAN_POINT ( 'NONE',  ( 0.7843704457339527591, 25.39269750000000059, -23.55949434567611078 ) ) ;
#16109=CARTESIAN_POINT ( 'NONE',  ( 19.51141091471011180, 29.75832250000000201, -1.622220754415315547 ) ) ;
#16126=CARTESIAN_POINT ( 'NONE',  ( 29.64606458365116737, 36.49567249999999774, -15.53894806404596096 ) ) ;
#16134=ADVANCED_FACE ( 'NONE', ( #6024 ), #19946, .F. ) ;
#16136=ORIENTED_EDGE ( 'NONE', *, *, #19951, .T. ) ;
#16138=EDGE_CURVE ( 'NONE', #3406, #4408, #11452, .T. ) ;
#16148=DIRECTION ( 'NONE',  ( 0.8558687090795834562, 0.000000000000000000, -0.5171931484643310650 ) ) ;
#16150=CARTESIAN_POINT ( 'NONE',  ( 8.781357490942916399, -7.547927499999999235, -18.85455479843708559 ) ) ;
#16160=ORIENTED_EDGE ( 'NONE', *, *, #8520, .F. ) ;
#16162=ORIENTED_EDGE ( 'NONE', *, *, #10458, .T. ) ;
#16163=DIRECTION ( 'NONE',  ( 0.2490110332224850509, 0.000000000000000000, -0.9685006480810792739 ) ) ;
#16167=ADVANCED_FACE ( 'NONE', ( #21725 ), #17179, .F. ) ;
#16172=VECTOR ( 'NONE', #11347, 1000.000000000000000 ) ;
#16262=VERTEX_POINT ( 'NONE', #7444 ) ;
#16267=EDGE_CURVE ( 'NONE', #17189, #8237, #4029, .T. ) ;
#16279=DIRECTION ( 'NONE',  ( -0.5087559856598098396, 0.000000000000000000, -0.8609107660235847392 ) ) ;
#16280=DIRECTION ( 'NONE',  ( -0.9685006480810790519, 0.000000000000000000, -0.2490110332224857170 ) ) ;
#16285=DIRECTION ( 'NONE',  ( 0.000000000000000000, -1.000000000000000000, 0.000000000000000000 ) ) ;
#16291=EDGE_CURVE ( 'NONE', #6123, #13945, #6619, .T. ) ;
#16325=DIRECTION ( 'NONE',  ( 0.2490110332224850231, 0.000000000000000000, -0.9685006480810791629 ) ) ;
#16326=LINE ( 'NONE', #15540, #1013 ) ;
#16328=VECTOR ( 'NONE', #11414, 1000.000000000000000 ) ;
#16358=DIRECTION ( 'NONE',  ( -0.5087559856598088404, 0.000000000000000000, -0.8609107660235851833 ) ) ;
#16361=DIRECTION ( 'NONE',  ( -0.2490110332224850509, 0.000000000000000000, 0.9685006480810792739 ) ) ;
#16367=( LENGTH_UNIT ( ) NAMED_UNIT ( * ) SI_UNIT ( .MILLI., .METRE. ) );
#16402=VECTOR ( 'NONE', #15820, 1000.000000000000000 ) ;
#16425=VERTEX_POINT ( 'NONE', #2799 ) ;
#16444=ORIENTED_EDGE ( 'NONE', *, *, #13736, .F. ) ;
#16452=CARTESIAN_POINT ( 'NONE',  ( 29.64606458365116737, 39.28205249999999893, -15.53894806404596096 ) ) ;
#16472=ORIENTED_EDGE ( 'NONE', *, *, #19795, .T. ) ;
#16482=ORIENTED_EDGE ( 'NONE', *, *, #19213, .T. ) ;
#16486=CYLINDRICAL_SURFACE ( 'NONE', #21114, 0.7950200000000005041 ) ;
#16489=DIRECTION ( 'NONE',  ( -0.2490110332224850231, 0.000000000000000000, 0.9685006480810791629 ) ) ;
#16492=CARTESIAN_POINT ( 'NONE',  ( 2.520748753591570690, -1.594802499999999013, -24.56335908395234924 ) ) ;
#16514=DIRECTION ( 'NONE',  ( 0.000000000000000000, 1.000000000000000000, 0.000000000000000000 ) ) ;
#16516=DIRECTION ( 'NONE',  ( -0.2490110332224850509, 0.000000000000000000, 0.9685006480810792739 ) ) ;
#16539=LINE ( 'NONE', #9668, #6292 ) ;
#16546=CARTESIAN_POINT ( 'NONE',  ( -5.863861779363051419, -1.594802499999999013, -34.80955303575778714 ) ) ;
#16551=DIRECTION ( 'NONE',  ( 0.000000000000000000, 1.000000000000000000, 0.000000000000000000 ) ) ;
#16565=VERTEX_POINT ( 'NONE', #19806 ) ;
#16566=ORIENTED_EDGE ( 'NONE', *, *, #11884, .T. ) ;
#16578=EDGE_CURVE ( 'NONE', #8349, #9790, #9847, .T. ) ;
#16585=EDGE_LOOP ( 'NONE', ( #13279, #15446, #6711, #18932, #7446 ) ) ;
#16589=ORIENTED_EDGE ( 'NONE', *, *, #20383, .T. ) ;
#16601=ORIENTED_EDGE ( 'NONE', *, *, #272, .F. ) ;
#16604=DIRECTION ( 'NONE',  ( -0.9685006480810791629, 0.000000000000000000, -0.2490110332224850231 ) ) ;
#16607=ORIENTED_EDGE ( 'NONE', *, *, #15235, .F. ) ;
#16610=ORIENTED_EDGE ( 'NONE', *, *, #13219, .T. ) ;
#16628=AXIS2_PLACEMENT_3D ( 'NONE', #6076, #12849, #19570 ) ;
#16629=ORIENTED_EDGE ( 'NONE', *, *, #157, .F. ) ;
#16641=LINE ( 'NONE', #21614, #16056 ) ;
#16650=EDGE_CURVE ( 'NONE', #16425, #1721, #18688, .T. ) ;
#16651=AXIS2_PLACEMENT_3D ( 'NONE', #20656, #328, #12505 ) ;
#16662=AXIS2_PLACEMENT_3D ( 'NONE', #18249, #4775, #19788 ) ;
#16671=VECTOR ( 'NONE', #15168, 1000.000000000000000 ) ;
#16711=DIRECTION ( 'NONE',  ( 0.000000000000000000, -1.000000000000000000, 0.000000000000000000 ) ) ;
#16720=AXIS2_PLACEMENT_3D ( 'NONE', #8092, #17956, #7886 ) ;
#16746=ORIENTED_EDGE ( 'NONE', *, *, #18458, .T. ) ;
#16767=VERTEX_POINT ( 'NONE', #11749 ) ;
#16785=FACE_OUTER_BOUND ( 'NONE', #6283, .T. ) ;
#16788=ORIENTED_EDGE ( 'NONE', *, *, #13005, .F. ) ;
#16798=ORIENTED_EDGE ( 'NONE', *, *, #7660, .T. ) ;
#16814=CARTESIAN_POINT ( 'NONE',  ( 29.15193331460030279, -6.752907499999998286, -13.61707959051006966 ) ) ;
#16820=ORIENTED_EDGE ( 'NONE', *, *, #2466, .T. ) ;
#16869=VERTEX_POINT ( 'NONE', #20675 ) ;
#16876=DIRECTION ( 'NONE',  ( -0.2490110332224850509, 0.000000000000000000, 0.9685006480810792739 ) ) ;
#16879=ORIENTED_EDGE ( 'NONE', *, *, #13318, .T. ) ;
#16888=CARTESIAN_POINT ( 'NONE',  ( 11.24737647850577993, 13.08957250000000094, -3.746985211334052046 ) ) ;
#16892=ORIENTED_EDGE ( 'NONE', *, *, #15235, .T. ) ;
#16901=ORIENTED_EDGE ( 'NONE', *, *, #5817, .T. ) ;
#16904=DIRECTION ( 'NONE',  ( 0.2490110332224850509, 0.000000000000000000, -0.9685006480810792739 ) ) ;
#16908=EDGE_CURVE ( 'NONE', #6167, #2495, #5650, .T. ) ;
#16938=AXIS2_PLACEMENT_3D ( 'NONE', #19018, #9293, #9179 ) ;
#16957=VECTOR ( 'NONE', #7782, 1000.000000000000114 ) ;
#16966=CIRCLE ( 'NONE', #7437, 0.7950200000000007261 ) ;
#16968=LINE ( 'NONE', #8890, #3183 ) ;
#16998=CARTESIAN_POINT ( 'NONE',  ( -3.845402119898529758, 2.373947500000000765, -31.39393985263922460 ) ) ;
#17001=ORIENTED_EDGE ( 'NONE', *, *, #8176, .T. ) ;
#17035=ORIENTED_EDGE ( 'NONE', *, *, #18833, .T. ) ;
#17041=CARTESIAN_POINT ( 'NONE',  ( 0.7843704457339527591, -1.594802499999999013, -23.55949434567611078 ) ) ;
#17049=FACE_OUTER_BOUND ( 'NONE', #20525, .T. ) ;
#17067=CARTESIAN_POINT ( 'NONE',  ( -7.949728765560771571, -1.265494433638964855, -34.47798802949893826 ) ) ;
#17084=EDGE_LOOP ( 'NONE', ( #17972, #17192, #14528, #12151 ) ) ;
#17093=ORIENTED_EDGE ( 'NONE', *, *, #1220, .T. ) ;
#17109=CARTESIAN_POINT ( 'NONE',  ( -2.234700160307072192, 3.961447500000001565, -24.80708529208898483 ) ) ;
#17111=CARTESIAN_POINT ( 'NONE',  ( 7.241402720468077092, 6.343967500000000648, -19.25049230170216319 ) ) ;
#17114=CARTESIAN_POINT ( 'NONE',  ( 1.291462649553421604, 34.12394749999999988, -20.78637864442907812 ) ) ;
#17122=EDGE_CURVE ( 'NONE', #1619, #16565, #13687, .T. ) ;
#17155=LINE ( 'NONE', #17041, #19690 ) ;
#17162=DIRECTION ( 'NONE',  ( 0.9685006480810790519, 0.000000000000000000, 0.2490110332224857170 ) ) ;
#17167=LINE ( 'NONE', #10311, #13 ) ;
#17178=CARTESIAN_POINT ( 'NONE',  ( 29.15193331460030279, 30.55334249999999940, -13.61707959051006966 ) ) ;
#17179=PLANE ( 'NONE',  #17470 ) ;
#17189=VERTEX_POINT ( 'NONE', #8909 ) ;
#17192=ORIENTED_EDGE ( 'NONE', *, *, #19993, .F. ) ;
#17201=ORIENTED_EDGE ( 'NONE', *, *, #14790, .T. ) ;
#17207=ADVANCED_BREP_SHAPE_REPRESENTATION ( '', ( #21013, #2234 ), #14439 ) ;
#17213=ORIENTED_EDGE ( 'NONE', *, *, #20412, .F. ) ;
#17216=CARTESIAN_POINT ( 'NONE',  ( 1.173720826352361080, 34.12394749999999988, -20.82884779549221577 ) ) ;
#17217=FACE_OUTER_BOUND ( 'NONE', #4229, .T. ) ;
#17244=CARTESIAN_POINT ( 'NONE',  ( 23.49608546833631451, 3.565842500000000914, -17.12016812500874252 ) ) ;
#17254=VERTEX_POINT ( 'NONE', #12238 ) ;
#17280=LINE ( 'NONE', #2125, #19104 ) ;
#17283=ORIENTED_EDGE ( 'NONE', *, *, #13454, .T. ) ;
#17289=ORIENTED_EDGE ( 'NONE', *, *, #10148, .T. ) ;
#17291=AXIS2_PLACEMENT_3D ( 'NONE', #5015, #8105, #11770 ) ;
#17295=CARTESIAN_POINT ( 'NONE',  ( 26.59920545652001067, 3.961447500000001565, -43.69048495915765074 ) ) ;
#17298=DIRECTION ( 'NONE',  ( 0.5087559856598092844, 0.000000000000000000, 0.8609107660235849613 ) ) ;
#17317=EDGE_CURVE ( 'NONE', #11827, #7489, #18534, .T. ) ;
#17322=VECTOR ( 'NONE', #3501, 1000.000000000000114 ) ;
#17324=DIRECTION ( 'NONE',  ( 0.5087559856598092844, 0.000000000000000000, 0.8609107660235849613 ) ) ;
#17326=CARTESIAN_POINT ( 'NONE',  ( 28.87608719841374949, -7.547927499999999235, -15.73691681567849976 ) ) ;
#17327=LINE ( 'NONE', #8916, #5535 ) ;
#17334=VECTOR ( 'NONE', #8161, 1000.000000000000000 ) ;
#17360=CIRCLE ( 'NONE', #19821, 0.7950200000000005041 ) ;
#17365=DIRECTION ( 'NONE',  ( -0.5087559856598089514, 0.000000000000000000, -0.8609107660235851833 ) ) ;
#17402=ORIENTED_EDGE ( 'NONE', *, *, #5899, .F. ) ;
#17417=FACE_OUTER_BOUND ( 'NONE', #2639, .T. ) ;
#17442=CARTESIAN_POINT ( 'NONE',  ( 17.34610635302146164, 13.08957250000000094, -18.70138818597152053 ) ) ;
#17460=VECTOR ( 'NONE', #2979, 1000.000000000000114 ) ;
#17462=ADVANCED_FACE ( 'NONE', ( #13033 ), #18105, .F. ) ;
#17470=AXIS2_PLACEMENT_3D ( 'NONE', #39, #6791, #2019 ) ;
#17472=DIRECTION ( 'NONE',  ( 0.9685006480810791629, -1.017240852913530016E-16, 0.2490110332224850231 ) ) ;
#17475=ORIENTED_EDGE ( 'NONE', *, *, #10458, .F. ) ;
#17479=EDGE_CURVE ( 'NONE', #16565, #17254, #6491, .T. ) ;
#17489=FACE_BOUND ( 'NONE', #20259, .T. ) ;
#17492=DIRECTION ( 'NONE',  ( 0.000000000000000000, -1.000000000000000000, 0.000000000000000000 ) ) ;
#17508=ORIENTED_EDGE ( 'NONE', *, *, #12874, .T. ) ;
#17541=DIRECTION ( 'NONE',  ( 0.8609107660235850723, 0.000000000000000000, -0.5087559856598092844 ) ) ;
#17551=EDGE_CURVE ( 'NONE', #9160, #16425, #21741, .T. ) ;
#17578=DIRECTION ( 'NONE',  ( 0.000000000000000000, 1.000000000000000000, 0.000000000000000000 ) ) ;
#17579=CARTESIAN_POINT ( 'NONE',  ( 0.2641497867371597752, 3.961447500000001565, -24.43980549416641068 ) ) ;
#17582=ORIENTED_EDGE ( 'NONE', *, *, #3484, .F. ) ;
#17586=CARTESIAN_POINT ( 'NONE',  ( -7.545238043312568088, -1.594802499999999013, -33.79351368943453338 ) ) ;
#17599=PRODUCT_DEFINITION_FORMATION_WITH_SPECIFIED_SOURCE ( 'ANY', '', #4744, .NOT_KNOWN. ) ;
#17602=DIRECTION ( 'NONE',  ( 0.2490110332224850509, 0.000000000000000000, -0.9685006480810792739 ) ) ;
#17611=ORIENTED_EDGE ( 'NONE', *, *, #2078, .T. ) ;
#17615=DIRECTION ( 'NONE',  ( -0.9685006480810791629, 0.000000000000000000, -0.2490110332224850231 ) ) ;
#17618=VECTOR ( 'NONE', #8984, 1000.000000000000114 ) ;
#17624=ORIENTED_EDGE ( 'NONE', *, *, #21261, .T. ) ;
#17644=DIRECTION ( 'NONE',  ( 1.000000000000000000, 0.000000000000000000, 0.000000000000000000 ) ) ;
#17648=CARTESIAN_POINT ( 'NONE',  ( -3.042350287543033716, 2.373947500000000765, -26.17378113315171007 ) ) ;
#17660=ORIENTED_EDGE ( 'NONE', *, *, #14790, .F. ) ;
#17669=ORIENTED_EDGE ( 'NONE', *, *, #13561, .F. ) ;
#17675=EDGE_LOOP ( 'NONE', ( #4935, #6665, #2157, #11848 ) ) ;
#17677=ORIENTED_EDGE ( 'NONE', *, *, #14508, .T. ) ;
#17696=CARTESIAN_POINT ( 'NONE',  ( 2.492193568723835462, 34.12394749999999988, -24.56873394466936134 ) ) ;
#17700=ADVANCED_FACE ( 'NONE', ( #19061 ), #5362, .F. ) ;
#17716=FACE_OUTER_BOUND ( 'NONE', #18099, .T. ) ;
#17754=VERTEX_POINT ( 'NONE', #20828 ) ;
#17755=ADVANCED_FACE ( 'NONE', ( #10790 ), #15893, .F. ) ;
#17759=ADVANCED_FACE ( 'NONE', ( #8898 ), #5697, .F. ) ;
#17762=FACE_OUTER_BOUND ( 'NONE', #15575, .T. ) ;
#17781=CARTESIAN_POINT ( 'NONE',  ( 29.64606458365116737, 1.975802500000001904, -15.53894806404596096 ) ) ;
#17786=EDGE_CURVE ( 'NONE', #2943, #21869, #8779, .T. ) ;
#17830=DIRECTION ( 'NONE',  ( 0.8609107660235850723, 0.000000000000000000, -0.5087559856598092844 ) ) ;
#17859=ORIENTED_EDGE ( 'NONE', *, *, #2788, .F. ) ;
#17871=CARTESIAN_POINT ( 'NONE',  ( 2.492193568723835462, -1.594802499999999013, -24.56873394466936134 ) ) ;
#17876=ORIENTED_EDGE ( 'NONE', *, *, #8346, .F. ) ;
#17885=ORIENTED_EDGE ( 'NONE', *, *, #1355, .F. ) ;
#17896=ORIENTED_EDGE ( 'NONE', *, *, #16039, .T. ) ;
#17935=CARTESIAN_POINT ( 'NONE',  ( 35.47639361272155867, -6.752907499999998286, -41.40807265590733977 ) ) ;
#17943=CIRCLE ( 'NONE', #18294, 0.7950200000000003930 ) ;
#17948=DIRECTION ( 'NONE',  ( -0.2490110332224850231, 0.000000000000000000, 0.9685006480810791629 ) ) ;
#17954=CARTESIAN_POINT ( 'NONE',  ( 8.505511374756364873, -6.752907499999998286, -20.97439202360551747 ) ) ;
#17956=DIRECTION ( 'NONE',  ( 0.2490110332224850509, 0.000000000000000000, -0.9685006480810792739 ) ) ;
#17963=ORIENTED_EDGE ( 'NONE', *, *, #13193, .F. ) ;
#17964=CARTESIAN_POINT ( 'NONE',  ( -6.268352501591477832, -0.7997824999999986195, -35.49402737582407497 ) ) ;
#17972=ORIENTED_EDGE ( 'NONE', *, *, #6381, .F. ) ;
#17975=VERTEX_POINT ( 'NONE', #21602 ) ;
#17994=ORIENTED_EDGE ( 'NONE', *, *, #13022, .T. ) ;
#17995=EDGE_CURVE ( 'NONE', #18464, #3406, #10949, .T. ) ;
#17997=ORIENTED_EDGE ( 'NONE', *, *, #18597, .T. ) ;
#18002=CARTESIAN_POINT ( 'NONE',  ( 1.923689137428217455, -0.9589899600121986056, -20.61772871637841220 ) ) ;
#18007=CARTESIAN_POINT ( 'NONE',  ( 1.532169971477637782, 5.548947500000001476, -20.71839214105750315 ) ) ;
#18013=ORIENTED_EDGE ( 'NONE', *, *, #12771, .T. ) ;
#18021=CARTESIAN_POINT ( 'NONE',  ( 4.936390548048069427, -1.594802499999999013, -19.84313358055101517 ) ) ;
#18064=AXIS2_PLACEMENT_3D ( 'NONE', #8839, #3773, #3659 ) ;
#18070=EDGE_CURVE ( 'NONE', #1480, #5927, #6351, .T. ) ;
#18071=CARTESIAN_POINT ( 'NONE',  ( -3.037751992662818257, 26.98019749999999917, -30.02724401157551526 ) ) ;
#18082=DIRECTION ( 'NONE',  ( 0.000000000000000000, 1.000000000000000000, 0.000000000000000000 ) ) ;
#18099=EDGE_LOOP ( 'NONE', ( #9513, #21511, #2718, #18383 ) ) ;
#18102=ORIENTED_EDGE ( 'NONE', *, *, #5294, .F. ) ;
#18104=AXIS2_PLACEMENT_3D ( 'NONE', #14018, #12337, #10683 ) ;
#18105=CYLINDRICAL_SURFACE ( 'NONE', #15221, 2.182812499999999378 ) ;
#18112=VERTEX_POINT ( 'NONE', #13428 ) ;
#18156=DIRECTION ( 'NONE',  ( -0.9685006480810791629, 0.000000000000000000, -0.2490110332224850509 ) ) ;
#18159=CARTESIAN_POINT ( 'NONE',  ( 8.781357490942916399, 40.07707250000000698, -18.85455479843708559 ) ) ;
#18161=DIRECTION ( 'NONE',  ( -0.9685006480810791629, 0.000000000000000000, -0.2490110332224850231 ) ) ;
#18169=DIRECTION ( 'NONE',  ( 0.000000000000000000, 1.000000000000000000, 0.000000000000000000 ) ) ;
#18177=EDGE_CURVE ( 'NONE', #20882, #21748, #19353, .T. ) ;
#18183=ORIENTED_EDGE ( 'NONE', *, *, #6158, .F. ) ;
#18192=VERTEX_POINT ( 'NONE', #11282 ) ;
#18199=EDGE_CURVE ( 'NONE', #1295, #14232, #9298, .T. ) ;
#18208=LINE ( 'NONE', #18300, #6366 ) ;
#18213=ORIENTED_EDGE ( 'NONE', *, *, #10493, .F. ) ;
#18214=CARTESIAN_POINT ( 'NONE',  ( 8.505511374756364873, 39.28205249999999893, -20.97439202360551747 ) ) ;
#18220=ADVANCED_FACE ( 'NONE', ( #14305 ), #21442, .T. ) ;
#18226=FACE_OUTER_BOUND ( 'NONE', #4870, .T. ) ;
#18241=EDGE_CURVE ( 'NONE', #18464, #12469, #9620, .T. ) ;
#18249=CARTESIAN_POINT ( 'NONE',  ( -1.427050033073577806, 26.98019749999999917, -23.44038945102687066 ) ) ;
#18294=AXIS2_PLACEMENT_3D ( 'NONE', #20783, #15841, #19344 ) ;
#18300=CARTESIAN_POINT ( 'NONE',  ( -0.8970842057359728061, 5.548947500000001476, -22.54358764576276286 ) ) ;
#18321=VECTOR ( 'NONE', #7169, 1000.000000000000114 ) ;
#18331=CARTESIAN_POINT ( 'NONE',  ( 8.505511374756364873, -1.985327499999998357, -20.97439202360551747 ) ) ;
#18338=ORIENTED_EDGE ( 'NONE', *, *, #13318, .F. ) ;
#18357=LINE ( 'NONE', #20225, #20871 ) ;
#18372=LINE ( 'NONE', #6981, #99 ) ;
#18381=VERTEX_POINT ( 'NONE', #3621 ) ;
#18383=ORIENTED_EDGE ( 'NONE', *, *, #4771, .F. ) ;
#18385=DIRECTION ( 'NONE',  ( -0.2490110332224850509, 0.000000000000000000, 0.9685006480810792739 ) ) ;
#18392=ORIENTED_EDGE ( 'NONE', *, *, #20646, .T. ) ;
#18397=ORIENTED_EDGE ( 'NONE', *, *, #7381, .F. ) ;
#18405=CARTESIAN_POINT ( 'NONE',  ( 0.7843704457339527591, 25.39269750000000059, -23.55949434567611078 ) ) ;
#18424=VECTOR ( 'NONE', #8800, 1000.000000000000114 ) ;
#18442=CARTESIAN_POINT ( 'NONE',  ( 23.00195419928544638, 28.96330250000000461, -15.19829965147284945 ) ) ;
#18451=VERTEX_POINT ( 'NONE', #18540 ) ;
#18458=EDGE_CURVE ( 'NONE', #8237, #16767, #5376, .T. ) ;
#18459=DIRECTION ( 'NONE',  ( 0.4564177847958862944, -0.8819931412481734068, 0.1173494972856528179 ) ) ;
#18464=VERTEX_POINT ( 'NONE', #10467 ) ;
#18491=CARTESIAN_POINT ( 'NONE',  ( -6.268352501591477832, -0.7997824999999986195, -35.49402737582407497 ) ) ;
#18524=ORIENTED_EDGE ( 'NONE', *, *, #2764, .F. ) ;
#18529=CARTESIAN_POINT ( 'NONE',  ( 1.670997140563193373, -1.594802499999999013, -22.76294857149378714 ) ) ;
#18534=LINE ( 'NONE', #3399, #17322 ) ;
#18540=CARTESIAN_POINT ( 'NONE',  ( 2.417820406479087580, 33.48813496001219647, -22.53959718991430350 ) ) ;
#18547=LINE ( 'NONE', #9416, #8168 ) ;
#18548=CARTESIAN_POINT ( 'NONE',  ( -1.427050033073577806, 25.39269750000000059, -23.44038945102687066 ) ) ;
#18554=ORIENTED_EDGE ( 'NONE', *, *, #4912, .T. ) ;
#18562=EDGE_CURVE ( 'NONE', #4289, #2298, #11968, .T. ) ;
#18594=DIRECTION ( 'NONE',  ( -0.2490110332224850231, 0.000000000000000000, 0.9685006480810791629 ) ) ;
#18597=EDGE_CURVE ( 'NONE', #8797, #2943, #720, .T. ) ;
#18606=CARTESIAN_POINT ( 'NONE',  ( -0.8970842057359728061, 5.548947500000001476, -22.54358764576276286 ) ) ;
#18623=VERTEX_POINT ( 'NONE', #2119 ) ;
#18643=CARTESIAN_POINT ( 'NONE',  ( 29.64606458365116737, 30.55334249999999940, -15.53894806404596096 ) ) ;
#18655=ORIENTED_EDGE ( 'NONE', *, *, #8520, .T. ) ;
#18664=CARTESIAN_POINT ( 'NONE',  ( -4.728951812473551897, 3.961447500000001565, -29.02782796843600011 ) ) ;
#18685=DIRECTION ( 'NONE',  ( -0.2490110332224849676, 0.000000000000000000, 0.9685006480810792739 ) ) ;
#18688=LINE ( 'NONE', #10, #11109 ) ;
#18697=VECTOR ( 'NONE', #16489, 1000.000000000000114 ) ;
#18699=CARTESIAN_POINT ( 'NONE',  ( -2.234700160307072192, 3.961447500000001565, -24.80708529208898483 ) ) ;
#18705=EDGE_CURVE ( 'NONE', #19184, #5628, #5433, .T. ) ;
#18712=EDGE_LOOP ( 'NONE', ( #3039, #10933, #19316, #12011, #15175, #12488, #6671, #16610, #21523, #8137, #7460, #10375, #19879, #3012, #17283, #1962, #10875, #12699 ) ) ;
#18726=AXIS2_PLACEMENT_3D ( 'NONE', #18851, #5470, #8458 ) ;
#18729=UNCERTAINTY_MEASURE_WITH_UNIT (LENGTH_MEASURE( 1.000000000000000082E-05 ), #8229, 'distance_accuracy_value', 'NONE');
#18730=LINE ( 'NONE', #12117, #12730 ) ;
#18736=DIRECTION ( 'NONE',  ( 0.000000000000000000, -1.000000000000000000, 0.000000000000000000 ) ) ;
#18745=CARTESIAN_POINT ( 'NONE',  ( 8.505511374756364873, 39.28205249999999893, -20.97439202360551747 ) ) ;
#18746=VERTEX_POINT ( 'NONE', #13190 ) ;
#18777=CIRCLE ( 'NONE', #2186, 1.587500000000001688 ) ;
#18781=EDGE_LOOP ( 'NONE', ( #15689, #2962, #9083, #15151 ) ) ;
#18813=DIRECTION ( 'NONE',  ( 0.000000000000000000, 1.000000000000000000, 0.000000000000000000 ) ) ;
#18824=CARTESIAN_POINT ( 'NONE',  ( 1.173720826352361080, -1.594802499999999013, -20.82884779549221577 ) ) ;
#18833=EDGE_CURVE ( 'NONE', #7807, #10315, #4549, .T. ) ;
#18839=ADVANCED_FACE ( 'NONE', ( #21564 ), #21449, .T. ) ;
#18845=AXIS2_PLACEMENT_3D ( 'NONE', #10751, #1000, #19893 ) ;
#18848=CARTESIAN_POINT ( 'NONE',  ( 8.505511374756364873, 6.343967500000000648, -20.97439202360551747 ) ) ;
#18851=CARTESIAN_POINT ( 'NONE',  ( 26.59920545652001067, 26.98019749999999917, -43.69048495915765074 ) ) ;
#18854=EDGE_CURVE ( 'NONE', #13538, #3590, #5998, .T. ) ;
#18859=VERTEX_POINT ( 'NONE', #4661 ) ;
#18870=LINE ( 'NONE', #7274, #13920 ) ;
#18871=DIRECTION ( 'NONE',  ( 0.000000000000000000, -1.000000000000000000, 0.000000000000000000 ) ) ;
#18884=ORIENTED_EDGE ( 'NONE', *, *, #6544, .T. ) ;
#18888=DIRECTION ( 'NONE',  ( 0.000000000000000000, 1.000000000000000000, 0.000000000000000000 ) ) ;
#18892=CARTESIAN_POINT ( 'NONE',  ( 8.011380105705496746, 24.59767750000000319, -19.05252355006962617 ) ) ;
#18893=EDGE_LOOP ( 'NONE', ( #19084, #16601, #11937, #8809 ) ) ;
#18897=DIRECTION ( 'NONE',  ( 0.8609107660235850723, 0.000000000000000000, -0.5087559856598092844 ) ) ;
#18898=VECTOR ( 'NONE', #4801, 1000.000000000000114 ) ;
#18904=VERTEX_POINT ( 'NONE', #11505 ) ;
#18932=ORIENTED_EDGE ( 'NONE', *, *, #6354, .T. ) ;
#18961=PLANE ( 'NONE',  #2973 ) ;
#18962=AXIS2_PLACEMENT_3D ( 'NONE', #11824, #13061, #3198 ) ;
#18978=ORIENTED_EDGE ( 'NONE', *, *, #19775, .T. ) ;
#18986=ORIENTED_EDGE ( 'NONE', *, *, #21577, .F. ) ;
#18999=ORIENTED_EDGE ( 'NONE', *, *, #16908, .T. ) ;
#19002=DIRECTION ( 'NONE',  ( 0.2490110332224850509, 0.000000000000000000, -0.9685006480810792739 ) ) ;
#19010=ORIENTED_EDGE ( 'NONE', *, *, #18177, .F. ) ;
#19018=CARTESIAN_POINT ( 'NONE',  ( -23.36909032872569014, 26.98019749999999917, -10.47372115209112842 ) ) ;
#19028=DIRECTION ( 'NONE',  ( -0.2490110332224850509, 0.000000000000000000, 0.9685006480810792739 ) ) ;
#19044=ORIENTED_EDGE ( 'NONE', *, *, #4185, .T. ) ;
#19049=DIRECTION ( 'NONE',  ( -0.5087559856598092844, 0.000000000000000000, -0.8609107660235849613 ) ) ;
#19061=FACE_OUTER_BOUND ( 'NONE', #3295, .T. ) ;
#19066=ORIENTED_EDGE ( 'NONE', *, *, #10687, .F. ) ;
#19074=ORIENTED_EDGE ( 'NONE', *, *, #19798, .T. ) ;
#19083=DIRECTION ( 'NONE',  ( -0.9685006480810790519, 0.000000000000000000, -0.2490110332224857170 ) ) ;
#19084=ORIENTED_EDGE ( 'NONE', *, *, #7381, .T. ) ;
#19086=DIRECTION ( 'NONE',  ( 0.2490110332224850509, 0.000000000000000000, -0.9685006480810792739 ) ) ;
#19104=VECTOR ( 'NONE', #4021, 1000.000000000000000 ) ;
#19119=ORIENTED_EDGE ( 'NONE', *, *, #13924, .T. ) ;
#19120=EDGE_LOOP ( 'NONE', ( #14595, #12716, #18884, #12143 ) ) ;
#19125=CIRCLE ( 'NONE', #13494, 1.587500000000001688 ) ;
#19132=CARTESIAN_POINT ( 'NONE',  ( 1.670997140563193373, 34.12394749999999988, -22.76294857149378714 ) ) ;
#19144=DIRECTION ( 'NONE',  ( 0.000000000000000000, 1.000000000000000000, 0.000000000000000000 ) ) ;
#19166=DIRECTION ( 'NONE',  ( 0.8558687090795832342, 0.000000000000000000, -0.5171931484643309540 ) ) ;
#19184=VERTEX_POINT ( 'NONE', #21000 ) ;
#19198=AXIS2_PLACEMENT_3D ( 'NONE', #5820, #514, #16015 ) ;
#19213=EDGE_CURVE ( 'NONE', #11803, #17975, #8948, .T. ) ;
#19231=ADVANCED_FACE ( 'NONE', ( #3877 ), #10503, .T. ) ;
#19236=LINE ( 'NONE', #17586, #7488 ) ;
#19251=CIRCLE ( 'NONE', #7255, 0.7950200000000003930 ) ;
#19278=DIRECTION ( 'NONE',  ( 0.000000000000000000, -1.000000000000000000, 0.000000000000000000 ) ) ;
#19284=CARTESIAN_POINT ( 'NONE',  ( -0.5435003404963313356, 26.98019749999999917, -25.80650133522849998 ) ) ;
#19288=ORIENTED_EDGE ( 'NONE', *, *, #7614, .F. ) ;
#19295=CARTESIAN_POINT ( 'NONE',  ( 1.663439973261383820, 33.32892749999999893, -22.73355581192510044 ) ) ;
#19298=CARTESIAN_POINT ( 'NONE',  ( 4.520836821130160388, -1.594802499999999013, -5.476444653012091379 ) ) ;
#19316=ORIENTED_EDGE ( 'NONE', *, *, #2598, .T. ) ;
#19324=CARTESIAN_POINT ( 'NONE',  ( 1.532169971477637782, 34.03012968715594866, -20.71839214105750315 ) ) ;
#19343=LINE ( 'NONE', #4211, #2376 ) ;
#19344=DIRECTION ( 'NONE',  ( -0.9685006480810790519, 0.000000000000000000, -0.2490110332224857170 ) ) ;
#19349=EDGE_CURVE ( 'NONE', #14236, #7630, #17360, .T. ) ;
#19353=LINE ( 'NONE', #4655, #18697 ) ;
#19376=CARTESIAN_POINT ( 'NONE',  ( -7.545238043312568088, 34.12394749999999988, -33.79351368943453338 ) ) ;
#19377=EDGE_CURVE ( 'NONE', #19979, #7768, #14381, .T. ) ;
#19383=FACE_OUTER_BOUND ( 'NONE', #10068, .T. ) ;
#19385=EDGE_CURVE ( 'NONE', #6167, #4861, #21207, .T. ) ;
#19388=LINE ( 'NONE', #2263, #16957 ) ;
#19398=ORIENTED_EDGE ( 'NONE', *, *, #19533, .T. ) ;
#19405=ORIENTED_EDGE ( 'NONE', *, *, #5282, .F. ) ;
#19413=DIRECTION ( 'NONE',  ( -0.2490110332224850231, 0.000000000000000000, 0.9685006480810791629 ) ) ;
#19420=ORIENTED_EDGE ( 'NONE', *, *, #20673, .T. ) ;
#19432=CARTESIAN_POINT ( 'NONE',  ( 1.445847263472733291, -1.594802499999999013, -6.267054683493481271 ) ) ;
#19482=AXIS2_PLACEMENT_3D ( 'NONE', #21784, #3122, #111 ) ;
#19487=EDGE_CURVE ( 'NONE', #2577, #3111, #9272, .T. ) ;
#19500=DIRECTION ( 'NONE',  ( 0.2490110332224850509, 0.000000000000000000, -0.9685006480810792739 ) ) ;
#19503=ORIENTED_EDGE ( 'NONE', *, *, #7732, .F. ) ;
#19504=LINE ( 'NONE', #12145, #12445 ) ;
#19517=CARTESIAN_POINT ( 'NONE',  ( 9.275488759993784527, 40.07707250000000698, -20.77642327197297689 ) ) ;
#19520=ORIENTED_EDGE ( 'NONE', *, *, #237, .T. ) ;
#19523=DIRECTION ( 'NONE',  ( -0.8609107660235850723, 0.000000000000000000, 0.5087559856598092844 ) ) ;
#19530=VECTOR ( 'NONE', #13212, 1000.000000000000000 ) ;
#19533=EDGE_CURVE ( 'NONE', #10280, #7768, #9924, .T. ) ;
#19534=LINE ( 'NONE', #11135, #5243 ) ;
#19538=ORIENTED_EDGE ( 'NONE', *, *, #8176, .F. ) ;
#19553=DIRECTION ( 'NONE',  ( -0.9685006480810790519, 0.000000000000000000, -0.2490110332224857170 ) ) ;
#19566=AXIS2_PLACEMENT_3D ( 'NONE', #14735, #4766, #9727 ) ;
#19570=DIRECTION ( 'NONE',  ( -0.5171931484643297328, 0.000000000000000000, -0.8558687090795841224 ) ) ;
#19603=CARTESIAN_POINT ( 'NONE',  ( -3.845402119898529758, 3.961447500000001565, -31.39393985263922460 ) ) ;
#19609=LINE ( 'NONE', #13326, #7851 ) ;
#19661=CIRCLE ( 'NONE', #10132, 0.7950200000000003930 ) ;
#19663=DIRECTION ( 'NONE',  ( 0.000000000000000000, -1.000000000000000000, 0.000000000000000000 ) ) ;
#19690=VECTOR ( 'NONE', #1665, 1000.000000000000114 ) ;
#19700=DIRECTION ( 'NONE',  ( 0.9685006480810792739, -0.000000000000000000, 0.2490110332224850509 ) ) ;
#19717=ORIENTED_EDGE ( 'NONE', *, *, #8346, .T. ) ;
#19721=DIRECTION ( 'NONE',  ( 0.000000000000000000, 1.000000000000000000, 0.000000000000000000 ) ) ;
#19731=ORIENTED_EDGE ( 'NONE', *, *, #3697, .F. ) ;
#19734=ORIENTED_EDGE ( 'NONE', *, *, #17317, .F. ) ;
#19736=AXIS2_PLACEMENT_3D ( 'NONE', #3936, #9110, #12457 ) ;
#19752=CIRCLE ( 'NONE', #13773, 0.7950200000000005041 ) ;
#19759=DIRECTION ( 'NONE',  ( -0.2490110332224850509, 0.000000000000000000, 0.9685006480810792739 ) ) ;
#19761=( NAMED_UNIT ( * ) SI_UNIT ( $, .STERADIAN. ) SOLID_ANGLE_UNIT ( ) );
#19764=VERTEX_POINT ( 'NONE', #12782 ) ;
#19770=EDGE_LOOP ( 'NONE', ( #10093, #9282, #13282, #4789 ) ) ;
#19775=EDGE_CURVE ( 'NONE', #7630, #14463, #19504, .T. ) ;
#19788=DIRECTION ( 'NONE',  ( -0.5087559856598088404, 0.000000000000000000, -0.8609107660235851833 ) ) ;
#19795=EDGE_CURVE ( 'NONE', #20725, #18904, #11681, .T. ) ;
#19796=VECTOR ( 'NONE', #5128, 1000.000000000000000 ) ;
#19798=EDGE_CURVE ( 'NONE', #14729, #10511, #15577, .T. ) ;
#19806=CARTESIAN_POINT ( 'NONE',  ( 8.505511374756364873, 34.51447250000000366, -20.97439202360551747 ) ) ;
#19813=CYLINDRICAL_SURFACE ( 'NONE', #16720, 3.174999999999999378 ) ;
#19818=LINE ( 'NONE', #8320, #18898 ) ;
#19821=AXIS2_PLACEMENT_3D ( 'NONE', #16048, #19759, #1091 ) ;
#19823=LINE ( 'NONE', #6565, #805 ) ;
#19826=EDGE_CURVE ( 'NONE', #513, #10018, #21248, .T. ) ;
#19836=ORIENTED_EDGE ( 'NONE', *, *, #15180, .F. ) ;
#19848=ORIENTED_EDGE ( 'NONE', *, *, #18199, .F. ) ;
#19875=CARTESIAN_POINT ( 'NONE',  ( 1.923689137428217455, 33.48813496001219647, -20.61772871637841220 ) ) ;
#19879=ORIENTED_EDGE ( 'NONE', *, *, #21851, .T. ) ;
#19880=ADVANCED_FACE ( 'NONE', ( #8920 ), #15698, .F. ) ;
#19882=EDGE_CURVE ( 'NONE', #16262, #15380, #20175, .T. ) ;
#19892=CARTESIAN_POINT ( 'NONE',  ( -3.042350287543033716, 28.56769750000000130, -26.17378113315171007 ) ) ;
#19893=DIRECTION ( 'NONE',  ( 0.9685006480810792739, 0.000000000000000000, 0.2490110332224850509 ) ) ;
#19921=CIRCLE ( 'NONE', #8639, 1.587499999999999911 ) ;
#19932=ORIENTED_EDGE ( 'NONE', *, *, #1220, .F. ) ;
#19946=CYLINDRICAL_SURFACE ( 'NONE', #21336, 1.587499999999998579 ) ;
#19951=EDGE_CURVE ( 'NONE', #14236, #20985, #19823, .T. ) ;
#19979=VERTEX_POINT ( 'NONE', #9548 ) ;
#19993=EDGE_CURVE ( 'NONE', #13945, #15355, #21479, .T. ) ;
#20020=EDGE_CURVE ( 'NONE', #10927, #2943, #19609, .T. ) ;
#20022=CARTESIAN_POINT ( 'NONE',  ( 0.7843704457339527591, 5.548947500000001476, -23.55949434567611078 ) ) ;
#20058=EDGE_LOOP ( 'NONE', ( #2435, #16482, #17896, #10841 ) ) ;
#20065=EDGE_CURVE ( 'NONE', #20863, #20753, #2933, .T. ) ;
#20081=CARTESIAN_POINT ( 'NONE',  ( -1.427050033073577806, 25.39269750000000059, -23.44038945102687066 ) ) ;
#20084=AXIS2_PLACEMENT_3D ( 'NONE', #21690, #11627, #6548 ) ;
#20105=CARTESIAN_POINT ( 'NONE',  ( 28.38195592936287781, 2.770822500000000854, -13.81504834214261024 ) ) ;
#20106=DIRECTION ( 'NONE',  ( 0.2490110332224850509, 0.000000000000000000, -0.9685006480810792739 ) ) ;
#20108=ORIENTED_EDGE ( 'NONE', *, *, #1355, .T. ) ;
#20116=DIRECTION ( 'NONE',  ( -0.2490110332224850509, 0.000000000000000000, 0.9685006480810792739 ) ) ;
#20123=CARTESIAN_POINT ( 'NONE',  ( 18.49922743714299855, 40.07707250000000698, -18.40490942454099965 ) ) ;
#20125=LINE ( 'NONE', #20022, #6472 ) ;
#20126=CARTESIAN_POINT ( 'NONE',  ( -3.845402119898529758, 3.961447500000001565, -31.39393985263922460 ) ) ;
#20146=CARTESIAN_POINT ( 'NONE',  ( -7.545238043312568088, -1.594802499999999013, -33.79351368943453338 ) ) ;
#20150=AXIS2_PLACEMENT_3D ( 'NONE', #17871, #18082, #7903 ) ;
#20163=VECTOR ( 'NONE', #9419, 1000.000000000000000 ) ;
#20175=CIRCLE ( 'NONE', #10669, 0.7950200000000005041 ) ;
#20176=CARTESIAN_POINT ( 'NONE',  ( 30.86636926788154156, 28.96330250000000461, -42.59335521360503662 ) ) ;
#20193=ORIENTED_EDGE ( 'NONE', *, *, #4537, .T. ) ;
#20211=CARTESIAN_POINT ( 'NONE',  ( -7.782183222554425406, 34.12394750000063937, -34.19446947475137932 ) ) ;
#20222=ORIENTED_EDGE ( 'NONE', *, *, #5621, .F. ) ;
#20225=CARTESIAN_POINT ( 'NONE',  ( 7.241402720468077092, 25.39269750000000059, -19.25049230170216319 ) ) ;
#20236=CARTESIAN_POINT ( 'NONE',  ( 29.15193331460030279, 1.975802500000001904, -13.61707959051006966 ) ) ;
#20243=AXIS2_PLACEMENT_3D ( 'NONE', #999, #7856, #3000 ) ;
#20259=EDGE_LOOP ( 'NONE', ( #19119, #6620, #3802, #13628 ) ) ;
#20276=CARTESIAN_POINT ( 'NONE',  ( 1.890011456816786062, -1.569666835661437165, -22.67530205718506053 ) ) ;
#20281=EDGE_CURVE ( 'NONE', #20634, #1619, #15560, .T. ) ;
#20289=DIRECTION ( 'NONE',  ( 0.000000000000000000, 1.000000000000000000, 0.000000000000000000 ) ) ;
#20306=EDGE_LOOP ( 'NONE', ( #6536, #17402, #14831, #9774, #9927 ) ) ;
#20330=FACE_OUTER_BOUND ( 'NONE', #16585, .T. ) ;
#20341=DIRECTION ( 'NONE',  ( -0.5087559856597484442, 0.000000000000000000, -0.8609107660236209325 ) ) ;
#20361=DIRECTION ( 'NONE',  ( -0.2490110332224850231, 0.000000000000000000, 0.9685006480810791629 ) ) ;
#20380=CARTESIAN_POINT ( 'NONE',  ( 1.998220421679061776, -1.515722362770699494, -22.64748046904500356 ) ) ;
#20383=EDGE_CURVE ( 'NONE', #16565, #18623, #10457, .T. ) ;
#20391=DIRECTION ( 'NONE',  ( 0.2490110332224850509, 0.000000000000000000, -0.9685006480810792739 ) ) ;
#20406=CARTESIAN_POINT ( 'NONE',  ( 18.49922743714299855, -7.547927499999999235, -18.40490942454099965 ) ) ;
#20412=EDGE_CURVE ( 'NONE', #5796, #14463, #20554, .T. ) ;
#20415=VERTEX_POINT ( 'NONE', #9010 ) ;
#20431=ORIENTED_EDGE ( 'NONE', *, *, #8537, .F. ) ;
#20447=DIRECTION ( 'NONE',  ( 0.000000000000000000, -1.000000000000000000, 0.000000000000000000 ) ) ;
#20504=CARTESIAN_POINT ( 'NONE',  ( 8.505511374756364873, 39.28205249999999893, -20.97439202360551747 ) ) ;
#20511=AXIS2_PLACEMENT_3D ( 'NONE', #15068, #4873, #6202 ) ;
#20525=EDGE_LOOP ( 'NONE', ( #5726, #15557, #14272, #2526, #13303, #15226, #16879, #21301, #6967, #17001, #13822, #6184, #18986, #49, #6498, #8562, #17289, #16746 ) ) ;
#20535=AXIS2_PLACEMENT_3D ( 'NONE', #11318, #6120, #9857 ) ;
#20542=ORIENTED_EDGE ( 'NONE', *, *, #6825, .T. ) ;
#20554=CIRCLE ( 'NONE', #18104, 3.174999999999998490 ) ;
#20567=FACE_OUTER_BOUND ( 'NONE', #10453, .T. ) ;
#20571=ADVANCED_FACE ( 'NONE', ( #7996 ), #7890, .T. ) ;
#20580=CARTESIAN_POINT ( 'NONE',  ( -5.863861779363051419, -1.594802499999999013, -34.80955303575778714 ) ) ;
#20582=CARTESIAN_POINT ( 'NONE',  ( 8.011380105705496746, 34.12394749999999988, -19.05252355006962617 ) ) ;
#20592=PRODUCT_DEFINITION ( 'UNKNOWN', '', #17599, #9214 ) ;
#20626=DIRECTION ( 'NONE',  ( 0.000000000000000000, 1.000000000000000000, 0.000000000000000000 ) ) ;
#20634=VERTEX_POINT ( 'NONE', #4551 ) ;
#20641=ORIENTED_EDGE ( 'NONE', *, *, #11698, .F. ) ;
#20646=EDGE_CURVE ( 'NONE', #16037, #14232, #8534, .T. ) ;
#20651=DIRECTION ( 'NONE',  ( 0.000000000000000000, -1.000000000000000000, 0.000000000000000000 ) ) ;
#20656=CARTESIAN_POINT ( 'NONE',  ( 35.47639361272155867, 1.975802500000001904, -41.40807265590733977 ) ) ;
#20657=DIRECTION ( 'NONE',  ( 0.000000000000000000, 1.000000000000000000, 0.000000000000000000 ) ) ;
#20659=AXIS2_PLACEMENT_3D ( 'NONE', #475, #7229, #18813 ) ;
#20673=EDGE_CURVE ( 'NONE', #1981, #21656, #8297, .T. ) ;
#20675=CARTESIAN_POINT ( 'NONE',  ( -5.536601939709260733, 3.961447500000001565, -30.39452380949970944 ) ) ;
#20682=EDGE_CURVE ( 'NONE', #19764, #1295, #11842, .T. ) ;
#20689=LINE ( 'NONE', #10763, #6754 ) ;
#20713=CIRCLE ( 'NONE', #11561, 0.7950200000000003930 ) ;
#20725=VERTEX_POINT ( 'NONE', #8621 ) ;
#20729=ADVANCED_FACE ( 'NONE', ( #15397 ), #222, .F. ) ;
#20738=DIRECTION ( 'NONE',  ( -0.8609107660235848503, 0.000000000000000000, 0.5087559856598096175 ) ) ;
#20747=ORIENTED_EDGE ( 'NONE', *, *, #5568, .F. ) ;
#20753=VERTEX_POINT ( 'NONE', #8726 ) ;
#20757=ORIENTED_EDGE ( 'NONE', *, *, #13005, .T. ) ;
#20762=LINE ( 'NONE', #5842, #16402 ) ;
#20769=DIRECTION ( 'NONE',  ( 0.2490110332224850231, 0.000000000000000000, -0.9685006480810791629 ) ) ;
#20783=CARTESIAN_POINT ( 'NONE',  ( 8.781357490942916399, -6.752907499999998286, -18.85455479843708559 ) ) ;
#20801=DIRECTION ( 'NONE',  ( -0.8558687090795832342, 0.000000000000000000, 0.5171931484643309540 ) ) ;
#20826=ORIENTED_EDGE ( 'NONE', *, *, #13219, .F. ) ;
#20828=CARTESIAN_POINT ( 'NONE',  ( -0.8970842057359728061, -1.594802499999999013, -22.54358764576276286 ) ) ;
#20838=AXIS2_PLACEMENT_3D ( 'NONE', #4053, #96, #1864 ) ;
#20863=VERTEX_POINT ( 'NONE', #15610 ) ;
#20865=ORIENTED_EDGE ( 'NONE', *, *, #5593, .F. ) ;
#20869=ADVANCED_FACE ( 'NONE', ( #5409 ), #2318, .F. ) ;
#20870=EDGE_CURVE ( 'NONE', #1216, #17975, #11723, .T. ) ;
#20871=VECTOR ( 'NONE', #18161, 1000.000000000000114 ) ;
#20874=DIRECTION ( 'NONE',  ( 0.9685006480810793850, 0.000000000000000000, 0.2490110332224848011 ) ) ;
#20882=VERTEX_POINT ( 'NONE', #15728 ) ;
#20899=AXIS2_PLACEMENT_3D ( 'NONE', #14036, #12360, #15370 ) ;
#20904=EDGE_CURVE ( 'NONE', #2298, #3111, #18777, .T. ) ;
#20935=CARTESIAN_POINT ( 'NONE',  ( -6.100806958593727458, -1.594802499992218126, -35.21050882107348912 ) ) ;
#20958=PLANE ( 'NONE',  #2523 ) ;
#20960=CARTESIAN_POINT ( 'NONE',  ( -7.949728765565600597, 33.32892749999999893, -34.47798802950714503 ) ) ;
#20968=DIRECTION ( 'NONE',  ( 0.5087559856598092844, 0.000000000000000000, 0.8609107660235849613 ) ) ;
#20985=VERTEX_POINT ( 'NONE', #4090 ) ;
#20990=EDGE_CURVE ( 'NONE', #1632, #14970, #14719, .T. ) ;
#20994=CARTESIAN_POINT ( 'NONE',  ( 2.520748753591570690, 34.12394749999999988, -24.56335908395234924 ) ) ;
#20996=PLANE ( 'NONE',  #6528 ) ;
#21000=CARTESIAN_POINT ( 'NONE',  ( 12.62386444219163373, 13.08957250000000094, -17.86660850434754266 ) ) ;
#21001=LINE ( 'NONE', #12392, #431 ) ;
#21013=MANIFOLD_SOLID_BREP ( 'Stock-MAS-676-1', #12795 ) ;
#21074=DIRECTION ( 'NONE',  ( 0.000000000000000000, -1.000000000000000000, 0.000000000000000000 ) ) ;
#21092=LINE ( 'NONE', #18002, #17460 ) ;
#21093=DIRECTION ( 'NONE',  ( 0.2490110332224850509, 0.000000000000000000, -0.9685006480810792739 ) ) ;
#21095=ORIENTED_EDGE ( 'NONE', *, *, #21707, .F. ) ;
#21097=FACE_OUTER_BOUND ( 'NONE', #10816, .T. ) ;
#21114=AXIS2_PLACEMENT_3D ( 'NONE', #20176, #16876, #1723 ) ;
#21155=VERTEX_POINT ( 'NONE', #17442 ) ;
#21178=CARTESIAN_POINT ( 'NONE',  ( -1.427050033073577806, 3.961447500000001565, -23.44038945102687066 ) ) ;
#21183=VERTEX_POINT ( 'NONE', #517 ) ;
#21188=VERTEX_POINT ( 'NONE', #7269 ) ;
#21192=ORIENTED_EDGE ( 'NONE', *, *, #19775, .F. ) ;
#21201=CYLINDRICAL_SURFACE ( 'NONE', #8299, 0.7950200000000005041 ) ;
#21207=LINE ( 'NONE', #18007, #420 ) ;
#21218=CYLINDRICAL_SURFACE ( 'NONE', #16628, 0.7950200000000022804 ) ;
#21222=VECTOR ( 'NONE', #17948, 1000.000000000000114 ) ;
#21244=AXIS2_PLACEMENT_3D ( 'NONE', #5757, #7842, #14289 ) ;
#21248=CIRCLE ( 'NONE', #788, 0.7950200000000005041 ) ;
#21251=AXIS2_PLACEMENT_3D ( 'NONE', #2541, #5848, #3879 ) ;
#21261=EDGE_CURVE ( 'NONE', #18192, #3590, #732, .T. ) ;
#21265=CARTESIAN_POINT ( 'NONE',  ( 1.663439973261383820, -0.7997824999999986195, -22.73355581192510044 ) ) ;
#21301=ORIENTED_EDGE ( 'NONE', *, *, #20870, .T. ) ;
#21321=CYLINDRICAL_SURFACE ( 'NONE', #2443, 0.7950200000000005041 ) ;
#21323=EDGE_LOOP ( 'NONE', ( #11095, #20431, #11682, #5845, #17885 ) ) ;
#21325=CARTESIAN_POINT ( 'NONE',  ( 13.11799571124250363, 19.43957250000000059, -19.78847697788343396 ) ) ;
#21336=AXIS2_PLACEMENT_3D ( 'NONE', #13016, #19523, #19721 ) ;
#21348=CARTESIAN_POINT ( 'NONE',  ( 8.505511374756364873, -1.594802499999999013, -20.97439202360551747 ) ) ;
#21367=DIRECTION ( 'NONE',  ( -0.8609107660235850723, 0.000000000000000000, 0.5087559856598092844 ) ) ;
#21371=ADVANCED_FACE ( 'NONE', ( #19383 ), #10668, .F. ) ;
#21377=VECTOR ( 'NONE', #9655, 1000.000000000000000 ) ;
#21379=ADVANCED_FACE ( 'NONE', ( #17417 ), #9098, .F. ) ;
#21400=ORIENTED_EDGE ( 'NONE', *, *, #20020, .F. ) ;
#21412=EDGE_LOOP ( 'NONE', ( #16566, #15239, #14716, #5727 ) ) ;
#21420=DIRECTION ( 'NONE',  ( 0.000000000000000000, 1.000000000000000000, 0.000000000000000000 ) ) ;
#21436=ORIENTED_EDGE ( 'NONE', *, *, #19349, .F. ) ;
#21442=CYLINDRICAL_SURFACE ( 'NONE', #12005, 1.587500000000000577 ) ;
#21443=DIRECTION ( 'NONE',  ( 0.2490110332224850509, 0.000000000000000000, -0.9685006480810792739 ) ) ;
#21449=CYLINDRICAL_SURFACE ( 'NONE', #8820, 0.7950200000000005041 ) ;
#21454=CARTESIAN_POINT ( 'NONE',  ( 29.64606458365116737, 30.55334249999999940, -15.53894806404596096 ) ) ;
#21471=CARTESIAN_POINT ( 'NONE',  ( 4.520836821130160388, 40.07707250000000698, -5.476444653012091379 ) ) ;
#21472=EDGE_CURVE ( 'NONE', #11803, #10917, #6003, .T. ) ;
#21479=LINE ( 'NONE', #17964, #14588 ) ;
#21490=CARTESIAN_POINT ( 'NONE',  ( 8.011380105705496746, 24.59767750000000319, -19.05252355006962617 ) ) ;
#21496=PRODUCT_DEFINITION_SHAPE ( 'NONE', 'NONE',  #20592 ) ;
#21507=ORIENTED_EDGE ( 'NONE', *, *, #15860, .T. ) ;
#21511=ORIENTED_EDGE ( 'NONE', *, *, #17122, .F. ) ;
#21523=ORIENTED_EDGE ( 'NONE', *, *, #13066, .T. ) ;
#21524=ADVANCED_FACE ( 'NONE', ( #11529 ), #12994, .F. ) ;
#21526=VECTOR ( 'NONE', #12964, 1000.000000000000114 ) ;
#21534=DIRECTION ( 'NONE',  ( 0.000000000000000000, 1.000000000000000000, 0.000000000000000000 ) ) ;
#21538=ORIENTED_EDGE ( 'NONE', *, *, #7682, .T. ) ;
#21552=ADVANCED_FACE ( 'NONE', ( #21587 ), #19813, .F. ) ;
#21564=FACE_OUTER_BOUND ( 'NONE', #1865, .T. ) ;
#21577=EDGE_CURVE ( 'NONE', #12681, #14041, #6447, .T. ) ;
#21579=ADVANCED_FACE ( 'NONE', ( #11100 ), #9539, .T. ) ;
#21587=FACE_OUTER_BOUND ( 'NONE', #21808, .T. ) ;
#21588=CIRCLE ( 'NONE', #12067, 1.587500000000001688 ) ;
#21602=CARTESIAN_POINT ( 'NONE',  ( -3.037751992662818257, 2.373947500000000765, -30.02724401157551526 ) ) ;
#21608=CARTESIAN_POINT ( 'NONE',  ( 8.011380105705496746, 39.28205249999999893, -19.05252355006962617 ) ) ;
#21610=EDGE_CURVE ( 'NONE', #19979, #20985, #5045, .T. ) ;
#21614=CARTESIAN_POINT ( 'NONE',  ( -3.037751992662818257, 2.373947500000000765, -30.02724401157551526 ) ) ;
#21619=CARTESIAN_POINT ( 'NONE',  ( 1.532169971477637782, 5.548947500000001476, -20.71839214105750315 ) ) ;
#21656=VERTEX_POINT ( 'NONE', #20236 ) ;
#21665=EDGE_CURVE ( 'NONE', #14041, #3111, #20125, .T. ) ;
#21671=CARTESIAN_POINT ( 'NONE',  ( -3.845402119898529758, 26.98019749999999917, -31.39393985263922460 ) ) ;
#21680=EDGE_CURVE ( 'NONE', #5667, #13538, #12852, .T. ) ;
#21690=CARTESIAN_POINT ( 'NONE',  ( 4.520836821130160388, 25.39269750000000059, -5.476444653012091379 ) ) ;
#21699=CARTESIAN_POINT ( 'NONE',  ( -7.949728765565600597, -0.7997824999999986195, -34.47798802950714503 ) ) ;
#21707=EDGE_CURVE ( 'NONE', #18746, #13538, #18372, .T. ) ;
#21725=FACE_OUTER_BOUND ( 'NONE', #20058, .T. ) ;
#21741=LINE ( 'NONE', #10227, #10567 ) ;
#21748=VERTEX_POINT ( 'NONE', #15188 ) ;
#21755=VERTEX_POINT ( 'NONE', #21800 ) ;
#21765=EDGE_LOOP ( 'NONE', ( #13813, #3836, #14499, #17859, #17994 ) ) ;
#21784=CARTESIAN_POINT ( 'NONE',  ( 25.66139003002496466, 2.770822500000000854, -0.04100069345253434805 ) ) ;
#21791=DIRECTION ( 'NONE',  ( -0.2490110332224850231, 0.000000000000000000, 0.9685006480810791629 ) ) ;
#21800=CARTESIAN_POINT ( 'NONE',  ( -7.545238043312568088, -1.594802499999999013, -33.79351368943453338 ) ) ;
#21808=EDGE_LOOP ( 'NONE', ( #19836, #2903, #13941, #1612 ) ) ;
#21840=DIRECTION ( 'NONE',  ( -0.2490110332224850231, 0.000000000000000000, 0.9685006480810791629 ) ) ;
#21851=EDGE_CURVE ( 'NONE', #16869, #18112, #7543, .T. ) ;
#21869=VERTEX_POINT ( 'NONE', #4113 ) ;
#21878=AXIS2_PLACEMENT_3D ( 'NONE', #8331, #18385, #9993 ) ;
#21880=CARTESIAN_POINT ( 'NONE',  ( -7.545238043312568088, 34.12394749999999988, -33.79351368943453338 ) ) ;
ENDSEC;
END-ISO-10303-21;
